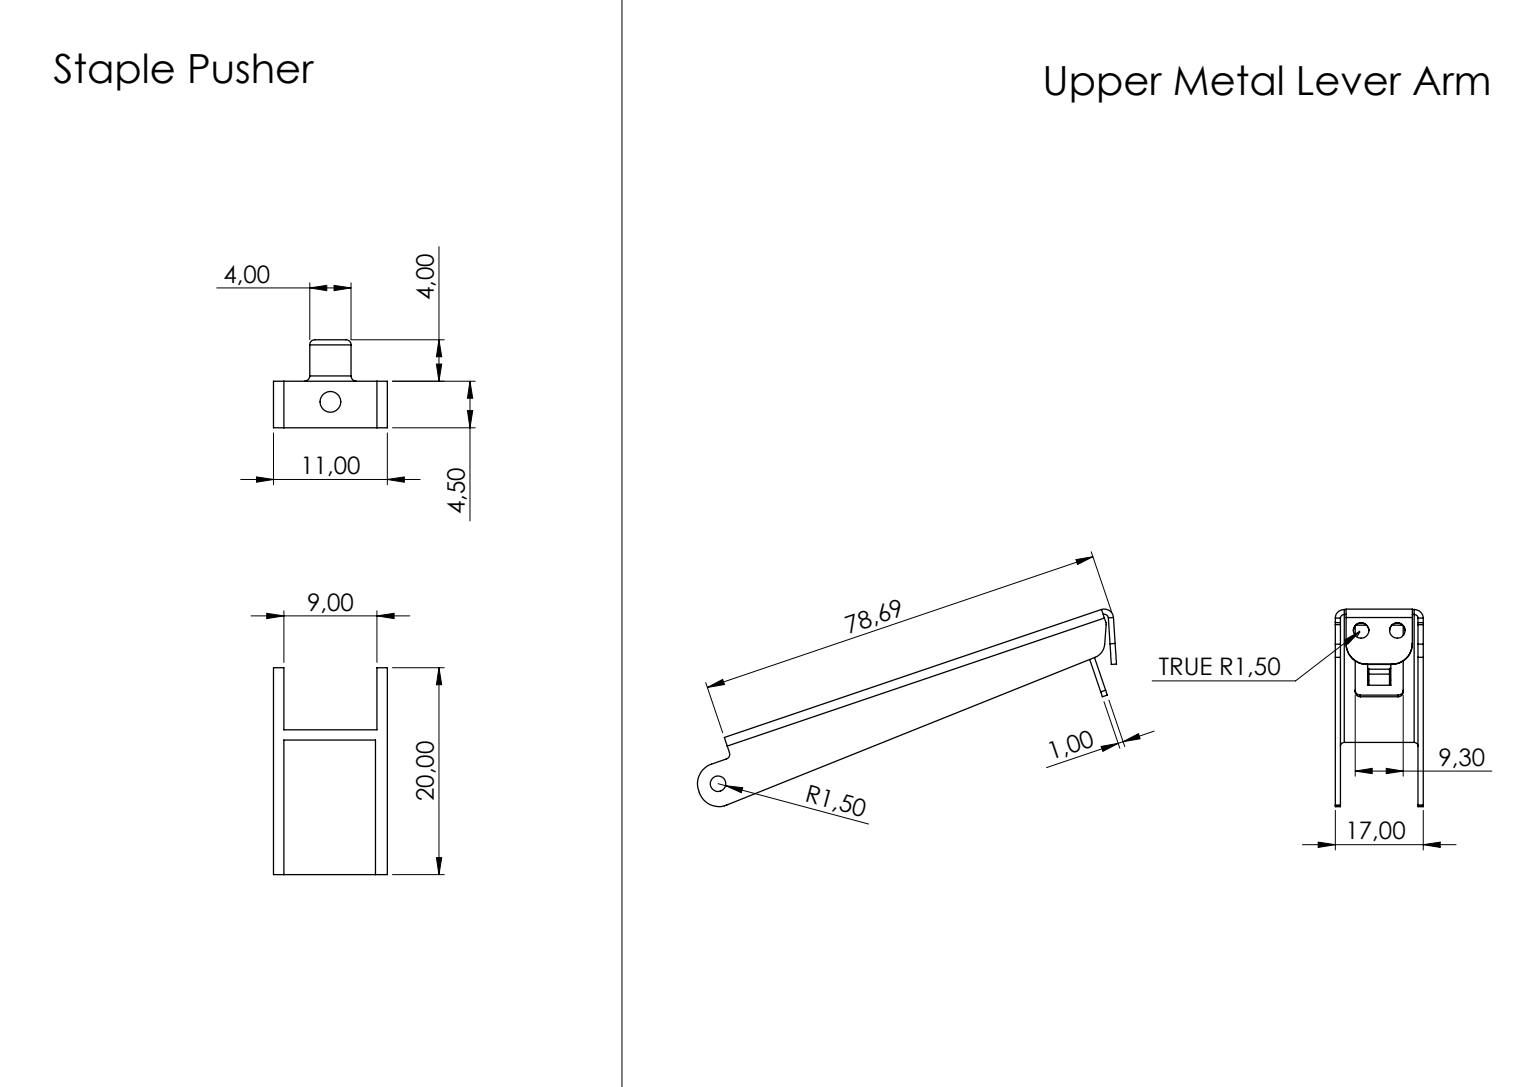
ISO-10303-21;
HEADER;
FILE_DESCRIPTION (('STEP AP214'),
    '1' );
FILE_NAME ('Upper Metal Lever Arm.step',
    '2026-10-06T10:23:46',
    ( '' ),
    ( '' ),
    'SwSTEP 2.0',
    'SolidWorks 2020',
    '' );
FILE_SCHEMA (( 'AUTOMOTIVE_DESIGN' ));
ENDSEC;

DATA;
#3=DIRECTION ( 'NONE',  ( -2.412663730047099099E-15, 0.8967398287344627850, 0.4425581086832399147 ) ) ;
#22=VERTEX_POINT ( 'NONE', #10978 ) ;
#26=DIRECTION ( 'NONE',  ( 1.327674326049719602E-15, -0.4425581086832399147, 0.8967398287344627850 ) ) ;
#34=ORIENTED_EDGE ( 'NONE', *, *, #8349, .T. ) ;
#35=DIRECTION ( 'NONE',  ( -1.000000000000000000, -3.091505625455828697E-15, -4.515976121274772923E-17 ) ) ;
#50=DIRECTION ( 'NONE',  ( 1.000000000000000000, 2.751104698760144965E-15, -1.228345504986737969E-16 ) ) ;
#58=VERTEX_POINT ( 'NONE', #8676 ) ;
#68=EDGE_LOOP ( 'NONE', ( #6538, #19929, #5268, #8723 ) ) ;
#84=CIRCLE ( 'NONE', #17364, 0.7500000000000006661 ) ;
#98=CARTESIAN_POINT ( 'NONE',  ( 29.81606138205697221, -3.227578639999851617, -4.500312080287595329 ) ) ;
#115=ORIENTED_EDGE ( 'NONE', *, *, #16759, .F. ) ;
#117=VECTOR ( 'NONE', #18081, 1000.000000000000000 ) ;
#122=AXIS2_PLACEMENT_3D ( 'NONE', #22603, #19127, #1077 ) ;
#180=VERTEX_POINT ( 'NONE', #7626 ) ;
#184=CARTESIAN_POINT ( 'NONE',  ( 31.91606138205697718, -5.022037326221728826, -5.474317061061731771 ) ) ;
#185=ORIENTED_EDGE ( 'NONE', *, *, #16638, .F. ) ;
#212=VECTOR ( 'NONE', #20996, 1000.000000000000000 ) ;
#213=AXIS2_PLACEMENT_3D ( 'NONE', #12528, #8134, #2696 ) ;
#214=CARTESIAN_POINT ( 'NONE',  ( 33.31606138205700773, -14.32738121993777192, 11.12118157620986558 ) ) ;
#224=ORIENTED_EDGE ( 'NONE', *, *, #10845, .T. ) ;
#227=DIRECTION ( 'NONE',  ( -1.000000000000000000, -2.999999999999999839E-15, 0.000000000000000000 ) ) ;
#238=ORIENTED_EDGE ( 'NONE', *, *, #7921, .F. ) ;
#248=CYLINDRICAL_SURFACE ( 'NONE', #25213, 0.7500000000000006661 ) ;
#274=EDGE_LOOP ( 'NONE', ( #318, #14239, #23744, #24928 ) ) ;
#279=ORIENTED_EDGE ( 'NONE', *, *, #5950, .F. ) ;
#290=ORIENTED_EDGE ( 'NONE', *, *, #14159, .F. ) ;
#298=ORIENTED_EDGE ( 'NONE', *, *, #19568, .F. ) ;
#308=VECTOR ( 'NONE', #6285, 1000.000000000000000 ) ;
#315=ORIENTED_EDGE ( 'NONE', *, *, #21706, .T. ) ;
#318=ORIENTED_EDGE ( 'NONE', *, *, #8973, .F. ) ;
#319=CYLINDRICAL_SURFACE ( 'NONE', #22266, 1.000000000000000888 ) ;
#322=MANIFOLD_SOLID_BREP ( 'NONE', #22112 ) ;
#345=VECTOR ( 'NONE', #23044, 1000.000000000000000 ) ;
#371=LINE ( 'NONE', #16872, #11443 ) ;
#386=CARTESIAN_POINT ( 'NONE',  ( 38.31606138205694378, 4.312150376739274371, 4.986822452676363149 ) ) ;
#387=VECTOR ( 'NONE', #11999, 1000.000000000000000 ) ;
#391=EDGE_CURVE ( 'NONE', #8203, #1835, #13926, .T. ) ;
#405=VECTOR ( 'NONE', #24075, 1000.000000000000000 ) ;
#424=PLANE ( 'NONE',  #3641 ) ;
#427=DIRECTION ( 'NONE',  ( 2.690219486203388234E-15, -0.8967398287344627850, -0.4425581086832399147 ) ) ;
#430=ADVANCED_FACE ( 'NONE', ( #17799 ), #14051, .T. ) ;
#433=CYLINDRICAL_SURFACE ( 'NONE', #4572, 0.7500000000000093259 ) ;
#436=PLANE ( 'NONE',  #12761 ) ;
#445=ORIENTED_EDGE ( 'NONE', *, *, #19266, .F. ) ;
#446=EDGE_CURVE ( 'NONE', #545, #18597, #371, .T. ) ;
#451=CARTESIAN_POINT ( 'NONE',  ( 33.80827534892208064, -18.91453975041207158, 24.37026150481227305 ) ) ;
#452=EDGE_LOOP ( 'NONE', ( #22783, #2146, #1836, #8004 ) ) ;
#459=CARTESIAN_POINT ( 'NONE',  ( 33.66606138205698073, -6.570990706613086374, -2.335727660491067503 ) ) ;
#480=DIRECTION ( 'NONE',  ( 1.327674326049719602E-15, -0.4425581086832399147, 0.8967398287344627850 ) ) ;
#481=AXIS2_PLACEMENT_3D ( 'NONE', #1514, #19059, #7211 ) ;
#483=( NAMED_UNIT ( * ) PLANE_ANGLE_UNIT ( ) SI_UNIT ( $, .RADIAN. ) );
#489=ORIENTED_EDGE ( 'NONE', *, *, #13595, .T. ) ;
#498=VECTOR ( 'NONE', #21104, 1000.000000000000114 ) ;
#502=LINE ( 'NONE', #5275, #212 ) ;
#509=EDGE_CURVE ( 'NONE', #23982, #20593, #22128, .T. ) ;
#523=EDGE_CURVE ( 'NONE', #15010, #2216, #1011, .T. ) ;
#535=ORIENTED_EDGE ( 'NONE', *, *, #15892, .T. ) ;
#545=VERTEX_POINT ( 'NONE', #10703 ) ;
#552=( GEOMETRIC_REPRESENTATION_CONTEXT ( 3 ) GLOBAL_UNCERTAINTY_ASSIGNED_CONTEXT ( ( #3328 ) ) GLOBAL_UNIT_ASSIGNED_CONTEXT ( ( #4972, #12369, #1089 ) ) REPRESENTATION_CONTEXT ( 'NONE', 'WORKASPACE' ) );
#559=VERTEX_POINT ( 'NONE', #14427 ) ;
#561=LINE ( 'NONE', #184, #3329 ) ;
#579=ADVANCED_FACE ( 'NONE', ( #24194 ), #4638, .F. ) ;
#594=EDGE_CURVE ( 'NONE', #6472, #12687, #11972, .T. ) ;
#598=ORIENTED_EDGE ( 'NONE', *, *, #10845, .F. ) ;
#604=ORIENTED_EDGE ( 'NONE', *, *, #15336, .F. ) ;
#611=LINE ( 'NONE', #20075, #6527 ) ;
#612=CARTESIAN_POINT ( 'NONE',  ( 46.81606138205702905, -23.83075694525939170, 32.63712566015296090 ) ) ;
#615=LINE ( 'NONE', #21762, #11077 ) ;
#623=EDGE_CURVE ( 'NONE', #5929, #22719, #8597, .T. ) ;
#628=LINE ( 'NONE', #17704, #1167 ) ;
#645=ORIENTED_EDGE ( 'NONE', *, *, #2860, .F. ) ;
#655=DIRECTION ( 'NONE',  ( -1.000000000000000000, -3.043523379167283935E-15, -1.423844882595663967E-16 ) ) ;
#656=LINE ( 'NONE', #2341, #117 ) ;
#658=EDGE_LOOP ( 'NONE', ( #5985, #10413, #8337, #20417 ) ) ;
#683=LINE ( 'NONE', #22085, #3287 ) ;
#709=CARTESIAN_POINT ( 'NONE',  ( 29.81606138205697221, -3.984974717493133145, -3.847356352999882656 ) ) ;
#710=FACE_OUTER_BOUND ( 'NONE', #21187, .T. ) ;
#714=EDGE_CURVE ( 'NONE', #8686, #3839, #3199, .T. ) ;
#733=DIRECTION ( 'NONE',  ( -1.000000000000000000, -2.999999999999999839E-15, 0.000000000000000000 ) ) ;
#748=ADVANCED_FACE ( 'NONE', ( #710 ), #20321, .F. ) ;
#749=ADVANCED_FACE ( 'NONE', ( #4354 ), #21994, .F. ) ;
#768=DIRECTION ( 'NONE',  ( 0.000000000000000000, -0.4425581086832400257, 0.8967398287344627850 ) ) ;
#776=LINE ( 'NONE', #24468, #17159 ) ;
#780=ORIENTED_EDGE ( 'NONE', *, *, #14281, .T. ) ;
#782=DIRECTION ( 'NONE',  ( -1.000000000000000000, -2.999999999999999839E-15, 0.000000000000000000 ) ) ;
#786=VERTEX_POINT ( 'NONE', #6157 ) ;
#809=CARTESIAN_POINT ( 'NONE',  ( 46.81606138205702194, -20.48383445069734066, 23.59578481461660004 ) ) ;
#834=LINE ( 'NONE', #10778, #14932 ) ;
#863=CARTESIAN_POINT ( 'NONE',  ( 31.91606138205697363, -3.929900956088018038, -7.102449327239662935 ) ) ;
#867=CARTESIAN_POINT ( 'NONE',  ( 42.96606138205694236, 5.208890205473748480, 5.429380561359602453 ) ) ;
#882=FACE_OUTER_BOUND ( 'NONE', #20497, .T. ) ;
#886=ADVANCED_FACE ( 'NONE', ( #3294 ), #4978, .F. ) ;
#896=ORIENTED_EDGE ( 'NONE', *, *, #24579, .T. ) ;
#914=VECTOR ( 'NONE', #23046, 1000.000000000000000 ) ;
#923=DIRECTION ( 'NONE',  ( 2.690219486203388234E-15, -0.8967398287344627850, -0.4425581086832399147 ) ) ;
#925=ORIENTED_EDGE ( 'NONE', *, *, #22452, .T. ) ;
#940=ORIENTED_EDGE ( 'NONE', *, *, #8964, .T. ) ;
#951=FACE_OUTER_BOUND ( 'NONE', #1705, .T. ) ;
#953=DIRECTION ( 'NONE',  ( -1.000000000000000000, -2.999999999999999839E-15, 0.000000000000000000 ) ) ;
#991=DIRECTION ( 'NONE',  ( -4.625929269271484533E-15, 0.8967398287344634511, 0.4425581086832385824 ) ) ;
#992=ORIENTED_EDGE ( 'NONE', *, *, #12189, .F. ) ;
#1011=LINE ( 'NONE', #8894, #24974 ) ;
#1017=EDGE_LOOP ( 'NONE', ( #16280, #22526, #11907, #24276 ) ) ;
#1029=LINE ( 'NONE', #18695, #10688 ) ;
#1034=ADVANCED_FACE ( 'NONE', ( #7294 ), #7553, .T. ) ;
#1043=ADVANCED_FACE ( 'NONE', ( #13603 ), #21202, .T. ) ;
#1047=LINE ( 'NONE', #4925, #6305 ) ;
#1052=DIRECTION ( 'NONE',  ( -2.011972697750612571E-15, 0.6595716529892353686, -0.7516416929448815898 ) ) ;
#1053=ADVANCED_FACE ( 'NONE', ( #5490 ), #11680, .T. ) ;
#1069=FACE_OUTER_BOUND ( 'NONE', #1734, .T. ) ;
#1071=ADVANCED_FACE ( 'NONE', ( #3542 ), #22998, .F. ) ;
#1072=EDGE_CURVE ( 'NONE', #3879, #7931, #5868, .T. ) ;
#1075=VERTEX_POINT ( 'NONE', #13231 ) ;
#1076=CARTESIAN_POINT ( 'NONE',  ( 41.06606138205700063, -13.51824891481308910, 37.72654391001022134 ) ) ;
#1077=DIRECTION ( 'NONE',  ( -4.625929269271484533E-15, 0.8967398287344634511, 0.4425581086832385824 ) ) ;
#1089=( NAMED_UNIT ( * ) SI_UNIT ( $, .STERADIAN. ) SOLID_ANGLE_UNIT ( ) );
#1105=ORIENTED_EDGE ( 'NONE', *, *, #4883, .F. ) ;
#1118=DIRECTION ( 'NONE',  ( 2.011972697750612571E-15, -0.6595716529892353686, 0.7516416929448815898 ) ) ;
#1135=( GEOMETRIC_REPRESENTATION_CONTEXT ( 3 ) GLOBAL_UNCERTAINTY_ASSIGNED_CONTEXT ( ( #17985 ) ) GLOBAL_UNIT_ASSIGNED_CONTEXT ( ( #4006, #12008, #23702 ) ) REPRESENTATION_CONTEXT ( 'NONE', 'WORKASPACE' ) );
#1139=LINE ( 'NONE', #6954, #7217 ) ;
#1156=VERTEX_POINT ( 'NONE', #2386 ) ;
#1157=AXIS2_PLACEMENT_3D ( 'NONE', #10550, #22012, #733 ) ;
#1160=ADVANCED_FACE ( 'NONE', ( #8080 ), #18126, .T. ) ;
#1164=ORIENTED_EDGE ( 'NONE', *, *, #19083, .T. ) ;
#1167=VECTOR ( 'NONE', #35, 1000.000000000000000 ) ;
#1170=DIRECTION ( 'NONE',  ( 1.180247624328911721E-15, -0.3934158747763039088, 0.9193606199277819524 ) ) ;
#1171=CARTESIAN_POINT ( 'NONE',  ( 37.31606138205699352, -10.61256217995208395, 37.48782943861662176 ) ) ;
#1185=LINE ( 'NONE', #1315, #3185 ) ;
#1204=ORIENTED_EDGE ( 'NONE', *, *, #24429, .F. ) ;
#1211=VECTOR ( 'NONE', #15036, 1000.000000000000000 ) ;
#1222=PRESENTATION_STYLE_ASSIGNMENT (( #4371 ) ) ;
#1232=DIRECTION ( 'NONE',  ( 1.000000000000000000, 2.999999999999999839E-15, 0.000000000000000000 ) ) ;
#1238=ORIENTED_EDGE ( 'NONE', *, *, #21451, .T. ) ;
#1254=DIRECTION ( 'NONE',  ( 1.000000000000000000, 3.194449454093636853E-15, 9.596449257708899394E-17 ) ) ;
#1255=EDGE_LOOP ( 'NONE', ( #21618, #11872, #14334, #19616 ) ) ;
#1258=DIRECTION ( 'NONE',  ( 1.327674326049719602E-15, -0.4425581086832399147, 0.8967398287344627850 ) ) ;
#1266=DIRECTION ( 'NONE',  ( -1.327674326049719602E-15, 0.4425581086832399147, -0.8967398287344627850 ) ) ;
#1269=CIRCLE ( 'NONE', #22659, 1.499999999999999778 ) ;
#1274=ADVANCED_FACE ( 'NONE', ( #3147 ), #15131, .T. ) ;
#1278=DIRECTION ( 'NONE',  ( -2.602085213965212219E-15, 0.8967398287344632291, 0.4425581086832389155 ) ) ;
#1285=AXIS2_PLACEMENT_3D ( 'NONE', #5753, #3813, #23012 ) ;
#1287=CYLINDRICAL_SURFACE ( 'NONE', #11276, 3.000000000000000000 ) ;
#1302=EDGE_CURVE ( 'NONE', #5803, #15873, #5351, .T. ) ;
#1315=CARTESIAN_POINT ( 'NONE',  ( 40.31606138205700773, -14.15704008206720843, 14.73030834591676808 ) ) ;
#1320=AXIS2_PLACEMENT_3D ( 'NONE', #1883, #23395, #7445 ) ;
#1344=AXIS2_PLACEMENT_3D ( 'NONE', #22886, #23011, #20710 ) ;
#1355=CARTESIAN_POINT ( 'NONE',  ( 29.81606138205696155, -0.7562224151693598406, -1.633662118351544734 ) ) ;
#1358=LINE ( 'NONE', #13469, #4116 ) ;
#1361=VECTOR ( 'NONE', #5593, 1000.000000000000000 ) ;
#1366=DIRECTION ( 'NONE',  ( 1.225631768639319301E-15, -0.4425581086832399147, 0.8967398287344627850 ) ) ;
#1368=EDGE_CURVE ( 'NONE', #9987, #15268, #10993, .T. ) ;
#1374=LINE ( 'NONE', #5377, #11185 ) ;
#1378=EDGE_CURVE ( 'NONE', #559, #12298, #7156, .T. ) ;
#1384=VECTOR ( 'NONE', #12923, 1000.000000000000000 ) ;
#1396=PLANE ( 'NONE',  #6605 ) ;
#1408=ORIENTED_EDGE ( 'NONE', *, *, #1499, .T. ) ;
#1409=PLANE ( 'NONE',  #22165 ) ;
#1411=DIRECTION ( 'NONE',  ( -1.000000000000000000, -3.091505625455828697E-15, -4.515976121274772923E-17 ) ) ;
#1436=DIRECTION ( 'NONE',  ( 2.792262043613788535E-15, -0.8967398287344627850, -0.4425581086832399147 ) ) ;
#1442=DIRECTION ( 'NONE',  ( -1.327674326049719602E-15, 0.4425581086832399147, -0.8967398287344627850 ) ) ;
#1443=ORIENTED_EDGE ( 'NONE', *, *, #14632, .F. ) ;
#1469=PLANE ( 'NONE',  #4053 ) ;
#1499=EDGE_CURVE ( 'NONE', #17110, #23130, #1965, .T. ) ;
#1514=CARTESIAN_POINT ( 'NONE',  ( 29.81606138205705037, -30.46100403034036219, 72.05704881431053366 ) ) ;
#1522=AXIS2_PLACEMENT_3D ( 'NONE', #25307, #23255, #13610 ) ;
#1527=CARTESIAN_POINT ( 'NONE',  ( 31.91606138205697363, -4.349482454670880571, -5.142398479549302515 ) ) ;
#1532=ORIENTED_EDGE ( 'NONE', *, *, #20926, .F. ) ;
#1535=EDGE_LOOP ( 'NONE', ( #11960, #24521, #19321, #10094 ) ) ;
#1571=EDGE_LOOP ( 'NONE', ( #19061, #21109, #19759, #17406 ) ) ;
#1578=CARTESIAN_POINT ( 'NONE',  ( 36.31606138205702194, -20.02093502212016318, 26.61211107664843212 ) ) ;
#1580=DIRECTION ( 'NONE',  ( -1.000000000000000000, -2.999999999999999839E-15, 0.000000000000000000 ) ) ;
#1594=LINE ( 'NONE', #7420, #2985 ) ;
#1599=CARTESIAN_POINT ( 'NONE',  ( 29.81606138205697221, -3.542416608809870304, -4.744096181734387407 ) ) ;
#1604=CARTESIAN_POINT ( 'NONE',  ( 29.81606138205696155, -0.7562224151693598406, -1.633662118351544734 ) ) ;
#1613=DIRECTION ( 'NONE',  ( 2.690219486203388234E-15, -0.8967398287344627850, -0.4425581086832399147 ) ) ;
#1615=FACE_OUTER_BOUND ( 'NONE', #21424, .T. ) ;
#1619=CIRCLE ( 'NONE', #4529, 0.7500000000000001110 ) ;
#1620=ORIENTED_EDGE ( 'NONE', *, *, #12683, .T. ) ;
#1631=CARTESIAN_POINT ( 'NONE',  ( 29.81606138205697221, -3.542416608809870304, -4.744096181734387407 ) ) ;
#1632=ORIENTED_EDGE ( 'NONE', *, *, #9283, .T. ) ;
#1638=VECTOR ( 'NONE', #3573, 1000.000000000000000 ) ;
#1639=EDGE_LOOP ( 'NONE', ( #23437, #3806, #3552, #24900, #2360, #12605 ) ) ;
#1640=DIRECTION ( 'NONE',  ( -2.312964634635742267E-15, 0.8967398287344634511, 0.4425581086832385824 ) ) ;
#1644=VERTEX_POINT ( 'NONE', #8551 ) ;
#1646=FACE_OUTER_BOUND ( 'NONE', #1724, .T. ) ;
#1647=CARTESIAN_POINT ( 'NONE',  ( 31.91606138205697363, -4.349482454670880571, -5.142398479549302515 ) ) ;
#1651=DIRECTION ( 'NONE',  ( -3.469446951953616555E-15, 0.8967398287344632291, 0.4425581086832389155 ) ) ;
#1659=ORIENTED_EDGE ( 'NONE', *, *, #10742, .T. ) ;
#1667=EDGE_CURVE ( 'NONE', #5253, #2986, #2770, .T. ) ;
#1695=ORIENTED_EDGE ( 'NONE', *, *, #19017, .F. ) ;
#1704=CARTESIAN_POINT ( 'NONE',  ( 45.81606138205697221, -3.984974717493084739, -3.847356352999882656 ) ) ;
#1705=EDGE_LOOP ( 'NONE', ( #1408, #19201, #23703, #1204 ) ) ;
#1706=CYLINDRICAL_SURFACE ( 'NONE', #23794, 1.750000000000001554 ) ;
#1716=CIRCLE ( 'NONE', #3370, 1.499999999999999778 ) ;
#1724=EDGE_LOOP ( 'NONE', ( #1878, #5691, #21493, #16540 ) ) ;
#1728=ADVANCED_FACE ( 'NONE', ( #2604 ), #23989, .F. ) ;
#1729=ORIENTED_EDGE ( 'NONE', *, *, #4047, .T. ) ;
#1734=EDGE_LOOP ( 'NONE', ( #185, #8919, #11633, #24570, #11697, #17570, #604, #9185, #598, #6119, #12537, #16413, #3459 ) ) ;
#1736=DIRECTION ( 'NONE',  ( -1.327674326049719602E-15, 0.4425581086832399147, -0.8967398287344627850 ) ) ;
#1754=DIRECTION ( 'NONE',  ( 3.965082230804126670E-15, -0.8967398287344626739, -0.4425581086832401922 ) ) ;
#1757=DIRECTION ( 'NONE',  ( 1.000000000000000000, 3.091505625455828697E-15, 4.515976121274772923E-17 ) ) ;
#1758=ADVANCED_FACE ( 'NONE', ( #19758 ), #5194, .F. ) ;
#1762=CARTESIAN_POINT ( 'NONE',  ( 34.81606138205697221, -3.103162021984047669, -5.046558096268735305 ) ) ;
#1768=LINE ( 'NONE', #21494, #19414 ) ;
#1778=ORIENTED_EDGE ( 'NONE', *, *, #18713, .F. ) ;
#1785=CIRCLE ( 'NONE', #13752, 3.999999999999997335 ) ;
#1809=DIRECTION ( 'NONE',  ( -1.292451913828718831E-15, 0.4425581086832399147, -0.8967398287344627850 ) ) ;
#1814=CARTESIAN_POINT ( 'NONE',  ( 46.81606138205706458, -34.13844651005145181, 70.48338531520533934 ) ) ;
#1820=EDGE_CURVE ( 'NONE', #24841, #1075, #6741, .T. ) ;
#1824=DIRECTION ( 'NONE',  ( -1.000000000000000000, -2.751104698760144965E-15, 1.228345504986737969E-16 ) ) ;
#1832=CARTESIAN_POINT ( 'NONE',  ( 45.81606138205697221, -3.542416608809821454, -4.744096181734387407 ) ) ;
#1835=VERTEX_POINT ( 'NONE', #11120 ) ;
#1836=ORIENTED_EDGE ( 'NONE', *, *, #15903, .T. ) ;
#1843=LINE ( 'NONE', #23311, #11133 ) ;
#1850=DIRECTION ( 'NONE',  ( 1.133678928659556219E-16, -0.4425581086832399147, 0.8967398287344627850 ) ) ;
#1852=DIRECTION ( 'NONE',  ( -2.690219486203387839E-15, 0.8967398287344625629, 0.4425581086832404143 ) ) ;
#1856=CARTESIAN_POINT ( 'NONE',  ( 40.31606138205699352, -10.61256217995207685, 37.48782943861662886 ) ) ;
#1878=ORIENTED_EDGE ( 'NONE', *, *, #18870, .F. ) ;
#1883=CARTESIAN_POINT ( 'NONE',  ( 41.81606138205696510, -1.316127829577467656, -4.808842309729777220 ) ) ;
#1885=LINE ( 'NONE', #25193, #4850 ) ;
#1888=ORIENTED_EDGE ( 'NONE', *, *, #14158, .T. ) ;
#1897=DIRECTION ( 'NONE',  ( 2.690219486203388234E-15, -0.8967398287344627850, -0.4425581086832399147 ) ) ;
#1904=CARTESIAN_POINT ( 'NONE',  ( 46.81606138205697221, -5.918777154956146980, -5.916875169744970187 ) ) ;
#1918=ORIENTED_EDGE ( 'NONE', *, *, #17611, .F. ) ;
#1923=CIRCLE ( 'NONE', #5236, 1.000000000000000888 ) ;
#1932=FACE_OUTER_BOUND ( 'NONE', #21271, .T. ) ;
#1933=DIRECTION ( 'NONE',  ( -1.327674326049719602E-15, 0.4425581086832399147, -0.8967398287344627850 ) ) ;
#1935=DIRECTION ( 'NONE',  ( -1.000000000000000000, -3.091505625455828697E-15, -4.515976121274772923E-17 ) ) ;
#1939=CARTESIAN_POINT ( 'NONE',  ( 42.96606138205694236, 5.208890205473748480, 5.429380561359602453 ) ) ;
#1959=VERTEX_POINT ( 'NONE', #23203 ) ;
#1965=CIRCLE ( 'NONE', #4849, 1.500000000000000222 ) ;
#1970=ORIENTED_EDGE ( 'NONE', *, *, #10049, .F. ) ;
#1976=DIRECTION ( 'NONE',  ( 1.000000000000000000, 2.751104698760144965E-15, -1.228345504986737969E-16 ) ) ;
#1978=DIRECTION ( 'NONE',  ( 2.341661252633485168E-15, -0.7516416929448815898, -0.6595716529892353686 ) ) ;
#1985=DIRECTION ( 'NONE',  ( -1.000000000000000000, -2.751104698760144965E-15, 1.228345504986737969E-16 ) ) ;
#1994=ORIENTED_EDGE ( 'NONE', *, *, #23549, .T. ) ;
#2000=AXIS2_PLACEMENT_3D ( 'NONE', #9286, #12766, #22537 ) ;
#2002=EDGE_CURVE ( 'NONE', #18170, #19403, #7283, .T. ) ;
#2014=LINE ( 'NONE', #25453, #14717 ) ;
#2022=LINE ( 'NONE', #21993, #11513 ) ;
#2024=CARTESIAN_POINT ( 'NONE',  ( 45.81606138205696510, -3.227578639999803212, -4.500312080287595329 ) ) ;
#2035=CARTESIAN_POINT ( 'NONE',  ( 29.81606138205697221, -3.984974717493133145, -3.847356352999882656 ) ) ;
#2038=EDGE_CURVE ( 'NONE', #7382, #23982, #19598, .T. ) ;
#2051=DIRECTION ( 'NONE',  ( -2.048868001712896742E-15, 0.6595716529892345914, -0.7516416929448823669 ) ) ;
#2062=EDGE_LOOP ( 'NONE', ( #19419, #10057, #1632, #10921 ) ) ;
#2073=DIRECTION ( 'NONE',  ( 1.000000000000000000, 3.091505625455829092E-15, 4.515976121274730398E-17 ) ) ;
#2075=DIRECTION ( 'NONE',  ( -1.000000000000000000, -2.827156040805656045E-15, 8.530177117963464484E-17 ) ) ;
#2077=LINE ( 'NONE', #2210, #20968 ) ;
#2082=CIRCLE ( 'NONE', #6616, 0.7500000000000006661 ) ;
#2086=EDGE_LOOP ( 'NONE', ( #18826, #3522, #1970, #2582 ) ) ;
#2089=AXIS2_PLACEMENT_3D ( 'NONE', #1604, #19524, #1985 ) ;
#2101=VERTEX_POINT ( 'NONE', #25378 ) ;
#2107=EDGE_LOOP ( 'NONE', ( #4877, #14552, #7560, #24954, #3602, #24123 ) ) ;
#2114=EDGE_LOOP ( 'NONE', ( #1105, #6601, #14755, #24647 ) ) ;
#2130=ADVANCED_FACE ( 'NONE', ( #15603 ), #23459, .F. ) ;
#2132=CARTESIAN_POINT ( 'NONE',  ( 33.31606138205700773, -14.32738121993777192, 11.12118157620986558 ) ) ;
#2135=ORIENTED_EDGE ( 'NONE', *, *, #6726, .F. ) ;
#2144=DIRECTION ( 'NONE',  ( -2.312964634635742267E-15, 0.8967398287344634511, 0.4425581086832385824 ) ) ;
#2146=ORIENTED_EDGE ( 'NONE', *, *, #8766, .T. ) ;
#2148=AXIS2_PLACEMENT_3D ( 'NONE', #23261, #1613, #5622 ) ;
#2165=AXIS2_PLACEMENT_3D ( 'NONE', #15015, #24281, #9111 ) ;
#2167=DIRECTION ( 'NONE',  ( 1.000000000000000000, 2.999999999999999839E-15, 0.000000000000000000 ) ) ;
#2172=VECTOR ( 'NONE', #15012, 1000.000000000000000 ) ;
#2179=DIRECTION ( 'NONE',  ( 3.469446951953614189E-15, -0.8967398287344635621, -0.4425581086832386379 ) ) ;
#2210=CARTESIAN_POINT ( 'NONE',  ( 30.81606138205705037, -30.65246816789535345, 72.44500581826353880 ) ) ;
#2216=VERTEX_POINT ( 'NONE', #5988 ) ;
#2220=LINE ( 'NONE', #15877, #21515 ) ;
#2234=CARTESIAN_POINT ( 'NONE',  ( 40.31606138205699352, -9.274586591516573719, 29.12776117315710067 ) ) ;
#2257=DIRECTION ( 'NONE',  ( -1.067465804653198538E-15, 0.4425581086832399147, -0.8967398287344627850 ) ) ;
#2268=FACE_OUTER_BOUND ( 'NONE', #23283, .T. ) ;
#2270=PLANE ( 'NONE',  #24587 ) ;
#2274=VERTEX_POINT ( 'NONE', #23112 ) ;
#2275=EDGE_CURVE ( 'NONE', #18597, #10242, #17586, .T. ) ;
#2285=LINE ( 'NONE', #98, #3817 ) ;
#2287=DIRECTION ( 'NONE',  ( -1.000000000000000000, -2.930207641762116835E-15, -1.414177847953724077E-16 ) ) ;
#2294=LINE ( 'NONE', #14284, #22983 ) ;
#2337=EDGE_LOOP ( 'NONE', ( #22884, #21057, #12205, #7070 ) ) ;
#2341=CARTESIAN_POINT ( 'NONE',  ( 46.81606138205697221, -4.349482454670835274, -5.142398479549302515 ) ) ;
#2344=ADVANCED_FACE ( 'NONE', ( #6238 ), #22329, .F. ) ;
#2360=ORIENTED_EDGE ( 'NONE', *, *, #4498, .F. ) ;
#2370=CARTESIAN_POINT ( 'NONE',  ( 43.31606138205695089, 3.741517323833267294, 2.753690589366190711 ) ) ;
#2379=EDGE_LOOP ( 'NONE', ( #2999, #17890, #19541, #15459 ) ) ;
#2386=CARTESIAN_POINT ( 'NONE',  ( 31.56606138205697576, -5.022037326221730602, -5.474317061061731771 ) ) ;
#2395=AXIS2_PLACEMENT_3D ( 'NONE', #14635, #3156, #12719 ) ;
#2399=DIRECTION ( 'NONE',  ( -4.625929269271484533E-15, 0.8967398287344634511, 0.4425581086832385824 ) ) ;
#2400=CARTESIAN_POINT ( 'NONE',  ( 30.81606138205697931, -5.918777154956195830, -5.916875169744970187 ) ) ;
#2429=ORIENTED_EDGE ( 'NONE', *, *, #14200, .T. ) ;
#2436=VECTOR ( 'NONE', #18030, 1000.000000000000000 ) ;
#2444=FACE_OUTER_BOUND ( 'NONE', #15215, .T. ) ;
#2449=CARTESIAN_POINT ( 'NONE',  ( 40.31606138205697221, -2.780187754385547105, -4.367921789353634843 ) ) ;
#2450=CARTESIAN_POINT ( 'NONE',  ( 40.56606138205696510, -1.522470315718718270, 0.9921758631592225708 ) ) ;
#2453=FACE_OUTER_BOUND ( 'NONE', #3327, .T. ) ;
#2478=ADVANCED_FACE ( 'NONE', ( #2483 ), #10355, .F. ) ;
#2483=FACE_OUTER_BOUND ( 'NONE', #24444, .T. ) ;
#2487=FACE_OUTER_BOUND ( 'NONE', #14398, .T. ) ;
#2512=ORIENTED_EDGE ( 'NONE', *, *, #4337, .T. ) ;
#2514=LINE ( 'NONE', #14380, #3833 ) ;
#2523=CARTESIAN_POINT ( 'NONE',  ( 33.66606138205698073, -6.672912525257930660, -0.4345143786932820218 ) ) ;
#2558=ADVANCED_FACE ( 'NONE', ( #17049 ), #14846, .F. ) ;
#2566=CARTESIAN_POINT ( 'NONE',  ( 45.81606138205707168, -38.42645682328033985, 63.90656833300437256 ) ) ;
#2567=AXIS2_PLACEMENT_3D ( 'NONE', #21845, #11433, #2257 ) ;
#2571=FACE_OUTER_BOUND ( 'NONE', #4228, .T. ) ;
#2582=ORIENTED_EDGE ( 'NONE', *, *, #4044, .F. ) ;
#2586=EDGE_CURVE ( 'NONE', #13895, #14345, #1185, .T. ) ;
#2604=FACE_OUTER_BOUND ( 'NONE', #7979, .T. ) ;
#2623=EDGE_CURVE ( 'NONE', #18307, #12298, #15934, .T. ) ;
#2625=VERTEX_POINT ( 'NONE', #23461 ) ;
#2649=ADVANCED_FACE ( 'NONE', ( #17680 ), #17299, .F. ) ;
#2670=DIRECTION ( 'NONE',  ( 1.000000000000000000, 3.021713267217945694E-15, 1.865775460081201246E-16 ) ) ;
#2696=DIRECTION ( 'NONE',  ( 2.690219486203388234E-15, -0.8967398287344627850, -0.4425581086832399147 ) ) ;
#2698=CARTESIAN_POINT ( 'NONE',  ( 44.71606138205697079, -3.195232061939673240, -6.457771442202879797 ) ) ;
#2704=CARTESIAN_POINT ( 'NONE',  ( 43.31606138205695089, 3.741517323833267294, 2.753690589366190711 ) ) ;
#2709=ORIENTED_EDGE ( 'NONE', *, *, #24840, .F. ) ;
#2722=DIRECTION ( 'NONE',  ( -1.047880217021202589E-15, 0.4425581086832399147, -0.8967398287344627850 ) ) ;
#2738=VERTEX_POINT ( 'NONE', #23593 ) ;
#2746=ORIENTED_EDGE ( 'NONE', *, *, #9299, .F. ) ;
#2748=DIRECTION ( 'NONE',  ( 2.690219486203388234E-15, -0.8967398287344627850, -0.4425581086832399147 ) ) ;
#2753=VECTOR ( 'NONE', #14063, 1000.000000000000000 ) ;
#2758=VERTEX_POINT ( 'NONE', #23205 ) ;
#2762=ADVANCED_FACE ( 'NONE', ( #15740 ), #5572, .T. ) ;
#2767=AXIS2_PLACEMENT_3D ( 'NONE', #14668, #24569, #10568 ) ;
#2770=CIRCLE ( 'NONE', #8983, 1.499999999999994005 ) ;
#2772=DIRECTION ( 'NONE',  ( 1.958867181863079949E-15, -0.6529557272876933549, -0.7573960774932753104 ) ) ;
#2775=CARTESIAN_POINT ( 'NONE',  ( 31.91606138205697363, -3.195232061939711432, -6.457771442202879797 ) ) ;
#2786=EDGE_CURVE ( 'NONE', #786, #13108, #25255, .T. ) ;
#2788=CARTESIAN_POINT ( 'NONE',  ( 31.56606138205697576, -4.349482454670882348, -5.142398479549302515 ) ) ;
#2796=CARTESIAN_POINT ( 'NONE',  ( 46.81606138205705037, -30.65246816789532502, 72.44500581826358143 ) ) ;
#2800=CARTESIAN_POINT ( 'NONE',  ( 44.71606138205697079, -3.854803714928911607, -5.706129749257958572 ) ) ;
#2805=CARTESIAN_POINT ( 'NONE',  ( 36.06606138205696510, -1.522470315718732037, 0.9921758631592225708 ) ) ;
#2823=CIRCLE ( 'NONE', #8627, 3.999999999999997335 ) ;
#2834=DIRECTION ( 'NONE',  ( 0.000000000000000000, -0.7516416929448823669, -0.6595716529892345914 ) ) ;
#2844=DIRECTION ( 'NONE',  ( 2.758081859783345370E-15, -0.9193606199277819524, -0.3934158747763039088 ) ) ;
#2847=VECTOR ( 'NONE', #13700, 1000.000000000000114 ) ;
#2860=EDGE_CURVE ( 'NONE', #16500, #2274, #4004, .T. ) ;
#2862=CARTESIAN_POINT ( 'NONE',  ( 33.31606138205695089, 3.741517323833236208, 2.753690589366190711 ) ) ;
#2868=ORIENTED_EDGE ( 'NONE', *, *, #23949, .T. ) ;
#2878=EDGE_CURVE ( 'NONE', #58, #2101, #22169, .T. ) ;
#2880=VERTEX_POINT ( 'NONE', #16357 ) ;
#2899=CARTESIAN_POINT ( 'NONE',  ( 34.81606138205696510, -1.316127829577488528, -4.808842309729777220 ) ) ;
#2905=CIRCLE ( 'NONE', #4160, 1.750000000000001554 ) ;
#2906=VERTEX_POINT ( 'NONE', #9952 ) ;
#2909=CARTESIAN_POINT ( 'NONE',  ( 46.81606138205697221, -5.022037326221683529, -5.474317061061731771 ) ) ;
#2918=DIRECTION ( 'NONE',  ( 2.690219486203388234E-15, -0.8967398287344627850, -0.4425581086832399147 ) ) ;
#2919=CARTESIAN_POINT ( 'NONE',  ( 29.81606138205706458, -34.13844651005150155, 70.48338531520533934 ) ) ;
#2923=CARTESIAN_POINT ( 'NONE',  ( 34.81606138205696510, -0.8482369431493941292, -3.067843137301039302 ) ) ;
#2932=ORIENTED_EDGE ( 'NONE', *, *, #16638, .T. ) ;
#2933=ORIENTED_EDGE ( 'NONE', *, *, #22167, .F. ) ;
#2959=ORIENTED_EDGE ( 'NONE', *, *, #22645, .T. ) ;
#2974=CIRCLE ( 'NONE', #15738, 0.7499999999999996669 ) ;
#2976=CARTESIAN_POINT ( 'NONE',  ( 43.31606138205700063, -14.32738121993773994, 11.12118157620986558 ) ) ;
#2984=DIRECTION ( 'NONE',  ( 1.327674326049719602E-15, -0.4425581086832399147, 0.8967398287344627850 ) ) ;
#2985=VECTOR ( 'NONE', #17332, 1000.000000000000000 ) ;
#2986=VERTEX_POINT ( 'NONE', #10083 ) ;
#2999=ORIENTED_EDGE ( 'NONE', *, *, #1378, .T. ) ;
#3031=CIRCLE ( 'NONE', #18669, 3.999999999999997335 ) ;
#3039=DIRECTION ( 'NONE',  ( -1.327674326049719602E-15, 0.4425581086832399147, -0.8967398287344627850 ) ) ;
#3041=( GEOMETRIC_REPRESENTATION_CONTEXT ( 3 ) GLOBAL_UNCERTAINTY_ASSIGNED_CONTEXT ( ( #24699 ) ) GLOBAL_UNIT_ASSIGNED_CONTEXT ( ( #5109, #483, #22135 ) ) REPRESENTATION_CONTEXT ( 'NONE', 'WORKASPACE' ) );
#3045=FACE_OUTER_BOUND ( 'NONE', #25037, .T. ) ;
#3063=ORIENTED_EDGE ( 'NONE', *, *, #3083, .T. ) ;
#3068=ORIENTED_EDGE ( 'NONE', *, *, #18672, .T. ) ;
#3072=LINE ( 'NONE', #5016, #12394 ) ;
#3074=DIRECTION ( 'NONE',  ( 1.000000000000000000, 2.602085213965208275E-15, 0.000000000000000000 ) ) ;
#3083=EDGE_CURVE ( 'NONE', #4595, #4703, #12650, .T. ) ;
#3089=EDGE_CURVE ( 'NONE', #2986, #5253, #14766, .T. ) ;
#3106=EDGE_CURVE ( 'NONE', #15655, #12192, #22421, .T. ) ;
#3107=ORIENTED_EDGE ( 'NONE', *, *, #18870, .T. ) ;
#3120=ORIENTED_EDGE ( 'NONE', *, *, #12244, .F. ) ;
#3122=CARTESIAN_POINT ( 'NONE',  ( 35.91606138205695942, 0.5799492015812600654, -3.145019409304214530 ) ) ;
#3134=ORIENTED_EDGE ( 'NONE', *, *, #5824, .F. ) ;
#3139=ORIENTED_EDGE ( 'NONE', *, *, #5484, .T. ) ;
#3141=CARTESIAN_POINT ( 'NONE',  ( 46.81606138205696510, -2.286980848581572356, -4.124514829577853980 ) ) ;
#3142=DIRECTION ( 'NONE',  ( 1.000000000000000000, 2.999999999999999839E-15, 0.000000000000000000 ) ) ;
#3144=CARTESIAN_POINT ( 'NONE',  ( 45.81606138205705037, -30.65246816789533213, 72.44500581826358143 ) ) ;
#3147=FACE_OUTER_BOUND ( 'NONE', #2379, .T. ) ;
#3148=ORIENTED_EDGE ( 'NONE', *, *, #12027, .F. ) ;
#3156=DIRECTION ( 'NONE',  ( -2.048868001712898319E-15, 0.6595716529892350355, -0.7516416929448821449 ) ) ;
#3166=ORIENTED_EDGE ( 'NONE', *, *, #10381, .T. ) ;
#3181=ORIENTED_EDGE ( 'NONE', *, *, #23246, .F. ) ;
#3185=VECTOR ( 'NONE', #8688, 1000.000000000000000 ) ;
#3190=EDGE_CURVE ( 'NONE', #22354, #4595, #18463, .T. ) ;
#3193=LINE ( 'NONE', #24443, #13204 ) ;
#3199=CIRCLE ( 'NONE', #12271, 1.500000000000000222 ) ;
#3202=EDGE_LOOP ( 'NONE', ( #12001, #23376, #21364, #9011 ) ) ;
#3204=DIRECTION ( 'NONE',  ( 1.000000000000000000, 2.611101091812726599E-15, -1.919289851541777660E-16 ) ) ;
#3217=VECTOR ( 'NONE', #23669, 1000.000000000000000 ) ;
#3223=CARTESIAN_POINT ( 'NONE',  ( 46.81606138205696510, -3.028410647649130816, 0.3252050635115383281 ) ) ;
#3250=EDGE_CURVE ( 'NONE', #8203, #1959, #4071, .T. ) ;
#3259=VECTOR ( 'NONE', #4287, 1000.000000000000000 ) ;
#3268=VERTEX_POINT ( 'NONE', #13655 ) ;
#3274=DIRECTION ( 'NONE',  ( -2.690219486203388234E-15, 0.8967398287344627850, 0.4425581086832399147 ) ) ;
#3287=VECTOR ( 'NONE', #16155, 1000.000000000000000 ) ;
#3294=FACE_OUTER_BOUND ( 'NONE', #4552, .T. ) ;
#3302=DIRECTION ( 'NONE',  ( 0.000000000000000000, -0.4425581086832348077, 0.8967398287344653385 ) ) ;
#3305=ORIENTED_EDGE ( 'NONE', *, *, #5617, .T. ) ;
#3313=VECTOR ( 'NONE', #7589, 1000.000000000000000 ) ;
#3319=CARTESIAN_POINT ( 'NONE',  ( 35.91606138205694521, 3.586515973360777654, -0.5067327973472466329 ) ) ;
#3325=DIRECTION ( 'NONE',  ( -1.000000000000000000, -2.999999999999999839E-15, 0.000000000000000000 ) ) ;
#3327=EDGE_LOOP ( 'NONE', ( #12452, #6895, #16216, #13853 ) ) ;
#3328=UNCERTAINTY_MEASURE_WITH_UNIT (LENGTH_MEASURE( 1.000000000000000082E-05 ), #4972, 'distance_accuracy_value', 'NONE');
#3329=VECTOR ( 'NONE', #7940, 1000.000000000000000 ) ;
#3355=ORIENTED_EDGE ( 'NONE', *, *, #9648, .T. ) ;
#3358=CARTESIAN_POINT ( 'NONE',  ( 33.31606138205697931, -6.570990706613088150, -2.335727660491067503 ) ) ;
#3367=EDGE_LOOP ( 'NONE', ( #25040, #9996, #22376, #20015 ) ) ;
#3369=LINE ( 'NONE', #1171, #6711 ) ;
#3370=AXIS2_PLACEMENT_3D ( 'NONE', #9033, #24457, #6829 ) ;
#3380=CIRCLE ( 'NONE', #10783, 1.750000000000001554 ) ;
#3386=ADVANCED_FACE ( 'NONE', ( #23808 ), #9923, .T. ) ;
#3407=EDGE_CURVE ( 'NONE', #2216, #7931, #18892, .T. ) ;
#3424=LINE ( 'NONE', #17090, #22197 ) ;
#3428=VECTOR ( 'NONE', #14336, 1000.000000000000000 ) ;
#3429=LINE ( 'NONE', #25165, #3725 ) ;
#3431=VERTEX_POINT ( 'NONE', #17780 ) ;
#3433=CARTESIAN_POINT ( 'NONE',  ( 40.31606138205697931, -5.528433326023618477, -4.448224773462933435 ) ) ;
#3442=EDGE_CURVE ( 'NONE', #58, #1644, #2294, .T. ) ;
#3444=AXIS2_PLACEMENT_3D ( 'NONE', #19832, #8112, #10052 ) ;
#3452=LINE ( 'NONE', #13629, #9000 ) ;
#3459=ORIENTED_EDGE ( 'NONE', *, *, #7029, .F. ) ;
#3463=LINE ( 'NONE', #6724, #9559 ) ;
#3486=EDGE_CURVE ( 'NONE', #21683, #5803, #615, .T. ) ;
#3491=DIRECTION ( 'NONE',  ( -2.011972697750612571E-15, 0.6595716529892353686, -0.7516416929448815898 ) ) ;
#3493=SURFACE_STYLE_FILL_AREA ( #19094 ) ;
#3495=FACE_OUTER_BOUND ( 'NONE', #2062, .T. ) ;
#3505=CARTESIAN_POINT ( 'NONE',  ( 44.71606138205695657, 0.5799492015812843793, -3.145019409304214530 ) ) ;
#3522=ORIENTED_EDGE ( 'NONE', *, *, #2038, .F. ) ;
#3526=CARTESIAN_POINT ( 'NONE',  ( 30.81606138205694378, 5.290470704224592424, -0.3848988112044732235 ) ) ;
#3538=CARTESIAN_POINT ( 'NONE',  ( 45.81606138205707168, -36.80651332587431313, 65.82119181171029254 ) ) ;
#3542=FACE_OUTER_BOUND ( 'NONE', #19197, .T. ) ;
#3552=ORIENTED_EDGE ( 'NONE', *, *, #1378, .F. ) ;
#3555=FACE_OUTER_BOUND ( 'NONE', #11528, .T. ) ;
#3561=CARTESIAN_POINT ( 'NONE',  ( 30.81606138205707168, -37.26069504592557990, 64.48189387429259511 ) ) ;
#3562=DIRECTION ( 'NONE',  ( -1.000000000000000000, -2.999999999999999839E-15, 0.000000000000000000 ) ) ;
#3565=AXIS2_PLACEMENT_3D ( 'NONE', #1856, #23499, #13357 ) ;
#3571=EDGE_CURVE ( 'NONE', #11586, #20804, #22520, .T. ) ;
#3573=DIRECTION ( 'NONE',  ( 1.000000000000000000, 2.751104698760144965E-15, -1.228345504986737969E-16 ) ) ;
#3589=CARTESIAN_POINT ( 'NONE',  ( 35.56606138205702194, -20.30191568716149675, 23.22716926412510219 ) ) ;
#3593=CARTESIAN_POINT ( 'NONE',  ( 45.81606138205707879, -39.99575152356564445, 63.13209164280871022 ) ) ;
#3602=ORIENTED_EDGE ( 'NONE', *, *, #20581, .F. ) ;
#3603=VECTOR ( 'NONE', #20223, 1000.000000000000000 ) ;
#3609=ORIENTED_EDGE ( 'NONE', *, *, #8349, .F. ) ;
#3612=SURFACE_STYLE_USAGE ( .BOTH. , #25107 ) ;
#3630=CARTESIAN_POINT ( 'NONE',  ( 46.81606138205707168, -38.13418765192403015, 68.51141129791366780 ) ) ;
#3639=AXIS2_PLACEMENT_3D ( 'NONE', #5279, #9032, #24576 ) ;
#3641=AXIS2_PLACEMENT_3D ( 'NONE', #13847, #4440, #7932 ) ;
#3662=VECTOR ( 'NONE', #11484, 1000.000000000000000 ) ;
#3664=FACE_OUTER_BOUND ( 'NONE', #19556, .T. ) ;
#3665=DIRECTION ( 'NONE',  ( -2.574571254471601357E-15, 0.8967398287344627850, 0.4425581086832399147 ) ) ;
#3666=DIRECTION ( 'NONE',  ( -1.000000000000000000, -2.999999999999999839E-15, 0.000000000000000000 ) ) ;
#3687=DIRECTION ( 'NONE',  ( 1.000000000000000000, 3.965082230804126670E-15, 0.000000000000000000 ) ) ;
#3695=AXIS2_PLACEMENT_3D ( 'NONE', #8825, #18351, #4943 ) ;
#3701=CARTESIAN_POINT ( 'NONE',  ( 30.81606138205706458, -34.54722833698622964, 70.28164373264664277 ) ) ;
#3705=CARTESIAN_POINT ( 'NONE',  ( 45.81606138205695800, -0.2703287878657676391, 1.505452687840413972 ) ) ;
#3709=CARTESIAN_POINT ( 'NONE',  ( 29.81606138205706458, -34.55876147768187678, 70.30501292735635843 ) ) ;
#3725=VECTOR ( 'NONE', #17094, 1000.000000000000000 ) ;
#3731=CARTESIAN_POINT ( 'NONE',  ( 41.81606138205696510, -1.975699482566714904, -4.057200616784870206 ) ) ;
#3743=CYLINDRICAL_SURFACE ( 'NONE', #22838, 1.000000000000000000 ) ;
#3747=PLANE ( 'NONE',  #8647 ) ;
#3753=ORIENTED_EDGE ( 'NONE', *, *, #23120, .F. ) ;
#3754=ADVANCED_FACE ( 'NONE', ( #25456, #7834, #17885 ), #5898, .T. ) ;
#3757=PRODUCT_CONTEXT ( 'NONE', #22302, 'mechanical' ) ;
#3772=ORIENTED_EDGE ( 'NONE', *, *, #6897, .T. ) ;
#3806=ORIENTED_EDGE ( 'NONE', *, *, #2623, .T. ) ;
#3813=DIRECTION ( 'NONE',  ( -1.000000000000000000, -2.999999999999999839E-15, 0.000000000000000000 ) ) ;
#3817=VECTOR ( 'NONE', #19823, 1000.000000000000000 ) ;
#3819=ORIENTED_EDGE ( 'NONE', *, *, #16170, .T. ) ;
#3824=ADVANCED_FACE ( 'NONE', ( #11597 ), #15319, .T. ) ;
#3833=VECTOR ( 'NONE', #19930, 1000.000000000000000 ) ;
#3839=VERTEX_POINT ( 'NONE', #13401 ) ;
#3851=CARTESIAN_POINT ( 'NONE',  ( 46.81606138205697221, -3.984974717493081187, -3.847356352999882656 ) ) ;
#3865=CIRCLE ( 'NONE', #7581, 1.000000000000011990 ) ;
#3875=EDGE_CURVE ( 'NONE', #21859, #2986, #23169, .T. ) ;
#3879=VERTEX_POINT ( 'NONE', #21248 ) ;
#3901=ADVANCED_FACE ( 'NONE', ( #1646 ), #9539, .T. ) ;
#3932=EDGE_CURVE ( 'NONE', #7931, #1075, #25345, .T. ) ;
#3934=CARTESIAN_POINT ( 'NONE',  ( 45.06606138205697221, -5.022037326221688858, -5.474317061061731771 ) ) ;
#3940=DIRECTION ( 'NONE',  ( -1.327674326049719602E-15, 0.4425581086832399147, -0.8967398287344627850 ) ) ;
#3978=ORIENTED_EDGE ( 'NONE', *, *, #13595, .F. ) ;
#3980=CARTESIAN_POINT ( 'NONE',  ( 31.56606138205707879, -39.09901169483120498, 63.57464975149190423 ) ) ;
#3987=CARTESIAN_POINT ( 'NONE',  ( 45.06606138205707879, -38.42645682328033985, 63.90656833300437256 ) ) ;
#3991=CARTESIAN_POINT ( 'NONE',  ( 29.81606138205709300, -43.53621639303161572, 70.30601027268440362 ) ) ;
#3996=EDGE_CURVE ( 'NONE', #7231, #14345, #8614, .T. ) ;
#4004=CIRCLE ( 'NONE', #18821, 0.7499999999999985567 ) ;
#4006=( LENGTH_UNIT ( ) NAMED_UNIT ( * ) SI_UNIT ( .MILLI., .METRE. ) );
#4007=ORIENTED_EDGE ( 'NONE', *, *, #14159, .T. ) ;
#4022=DIRECTION ( 'NONE',  ( -2.574571254471601357E-15, 0.8967398287344627850, 0.4425581086832399147 ) ) ;
#4024=DIRECTION ( 'NONE',  ( 0.000000000000000000, 0.6595716529892349245, -0.7516416929448820339 ) ) ;
#4033=ORIENTED_EDGE ( 'NONE', *, *, #3407, .T. ) ;
#4044=EDGE_CURVE ( 'NONE', #20593, #18694, #9123, .T. ) ;
#4047=EDGE_CURVE ( 'NONE', #13742, #19743, #12850, .T. ) ;
#4053=AXIS2_PLACEMENT_3D ( 'NONE', #3526, #3274, #1580 ) ;
#4071=CIRCLE ( 'NONE', #23396, 1.000000000000000000 ) ;
#4080=AXIS2_PLACEMENT_3D ( 'NONE', #20303, #18610, #953 ) ;
#4088=VECTOR ( 'NONE', #14601, 1000.000000000000000 ) ;
#4098=CARTESIAN_POINT ( 'NONE',  ( 41.06606138205700063, -13.51824891481308910, 37.72654391001022134 ) ) ;
#4103=ORIENTED_EDGE ( 'NONE', *, *, #5014, .F. ) ;
#4107=ORIENTED_EDGE ( 'NONE', *, *, #1499, .F. ) ;
#4113=CARTESIAN_POINT ( 'NONE',  ( 36.31606138205696510, -2.780187754385557319, -4.367921789353634843 ) ) ;
#4116=VECTOR ( 'NONE', #3665, 1000.000000000000000 ) ;
#4118=DIRECTION ( 'NONE',  ( 0.000000000000000000, -0.4425581086832385824, 0.8967398287344634511 ) ) ;
#4122=DIRECTION ( 'NONE',  ( 2.792262043613788535E-15, -0.8967398287344627850, -0.4425581086832399147 ) ) ;
#4129=CARTESIAN_POINT ( 'NONE',  ( 34.81606138205695800, -0.1886652901601799104, -3.819484830245897911 ) ) ;
#4136=CARTESIAN_POINT ( 'NONE',  ( 46.81606138205697221, -3.542416608809818346, -4.744096181734387407 ) ) ;
#4157=LINE ( 'NONE', #8275, #20131 ) ;
#4160=AXIS2_PLACEMENT_3D ( 'NONE', #24016, #12704, #6391 ) ;
#4167=AXIS2_PLACEMENT_3D ( 'NONE', #19645, #15654, #9368 ) ;
#4172=CYLINDRICAL_SURFACE ( 'NONE', #10075, 1.000000000000000888 ) ;
#4191=VERTEX_POINT ( 'NONE', #12193 ) ;
#4193=ORIENTED_EDGE ( 'NONE', *, *, #8608, .T. ) ;
#4207=EDGE_CURVE ( 'NONE', #15653, #24211, #683, .T. ) ;
#4215=EDGE_CURVE ( 'NONE', #22990, #1075, #18114, .T. ) ;
#4218=ORIENTED_EDGE ( 'NONE', *, *, #23120, .T. ) ;
#4220=DIRECTION ( 'NONE',  ( -2.792262043613788535E-15, 0.8967398287344627850, 0.4425581086832399147 ) ) ;
#4221=AXIS2_PLACEMENT_3D ( 'NONE', #18915, #4872, #1258 ) ;
#4228=EDGE_LOOP ( 'NONE', ( #18609, #19894, #8711, #23244 ) ) ;
#4229=CARTESIAN_POINT ( 'NONE',  ( 40.56606138205696510, -1.965028424401960461, 1.888915691893686244 ) ) ;
#4231=ADVANCED_FACE ( 'NONE', ( #4449 ), #436, .T. ) ;
#4238=EDGE_CURVE ( 'NONE', #12829, #6472, #1619, .T. ) ;
#4242=CIRCLE ( 'NONE', #21156, 1.500000000000000222 ) ;
#4248=ADVANCED_FACE ( 'NONE', ( #12578 ), #10372, .F. ) ;
#4253=DIRECTION ( 'NONE',  ( -2.792262043613788535E-15, 0.8967398287344627850, 0.4425581086832398592 ) ) ;
#4255=ORIENTED_EDGE ( 'NONE', *, *, #24177, .T. ) ;
#4261=ORIENTED_EDGE ( 'NONE', *, *, #5484, .F. ) ;
#4262=AXIS2_PLACEMENT_3D ( 'NONE', #18101, #10114, #12305 ) ;
#4273=CARTESIAN_POINT ( 'NONE',  ( 29.81606138205707168, -36.80651332587436286, 65.82119181171029254 ) ) ;
#4287=DIRECTION ( 'NONE',  ( -2.792262043613788535E-15, 0.8967398287344627850, 0.4425581086832399147 ) ) ;
#4295=ORIENTED_EDGE ( 'NONE', *, *, #23106, .T. ) ;
#4296=CARTESIAN_POINT ( 'NONE',  ( 30.81606138205707524, -38.42645682328038248, 63.90656833300437256 ) ) ;
#4297=AXIS2_PLACEMENT_3D ( 'NONE', #15497, #7785, #7912 ) ;
#4310=DIRECTION ( 'NONE',  ( -1.000000000000000000, -2.999999999999999839E-15, 0.000000000000000000 ) ) ;
#4312=DIRECTION ( 'NONE',  ( 1.327674326049719602E-15, -0.4425581086832399147, 0.8967398287344627850 ) ) ;
#4325=ORIENTED_EDGE ( 'NONE', *, *, #4714, .T. ) ;
#4326=DIRECTION ( 'NONE',  ( -1.000000000000000000, -2.999999999999999839E-15, 0.000000000000000000 ) ) ;
#4329=DIRECTION ( 'NONE',  ( -1.327674326049719602E-15, 0.4425581086832399147, -0.8967398287344627850 ) ) ;
#4337=EDGE_CURVE ( 'NONE', #23131, #16929, #20031, .T. ) ;
#4346=DIRECTION ( 'NONE',  ( 1.000000000000000000, 2.999999999999999839E-15, 0.000000000000000000 ) ) ;
#4349=DIRECTION ( 'NONE',  ( -1.000000000000000000, -2.999999999999999839E-15, 0.000000000000000000 ) ) ;
#4354=FACE_OUTER_BOUND ( 'NONE', #14705, .T. ) ;
#4362=CARTESIAN_POINT ( 'NONE',  ( 45.81606138205696510, -3.028410647649132592, 0.3252050635115383281 ) ) ;
#4364=CARTESIAN_POINT ( 'NONE',  ( 46.81606138205701484, -19.34838015056928029, 26.94402965816085072 ) ) ;
#4367=CARTESIAN_POINT ( 'NONE',  ( 40.31606138205701484, -18.91453975041205382, 24.37026150481227305 ) ) ;
#4371=SURFACE_STYLE_USAGE ( .BOTH. , #16693 ) ;
#4390=CARTESIAN_POINT ( 'NONE',  ( 46.81606138205695800, -0.7562224151693112129, -1.633662118351544734 ) ) ;
#4404=LINE ( 'NONE', #20115, #5273 ) ;
#4417=ORIENTED_EDGE ( 'NONE', *, *, #8727, .T. ) ;
#4419=CYLINDRICAL_SURFACE ( 'NONE', #7963, 1.750000000000001998 ) ;
#4424=CARTESIAN_POINT ( 'NONE',  ( 44.71606138205697079, -3.854803714928911607, -5.706129749257958572 ) ) ;
#4430=EDGE_CURVE ( 'NONE', #4703, #9931, #13981, .T. ) ;
#4434=AXIS2_PLACEMENT_3D ( 'NONE', #21593, #3940, #21713 ) ;
#4440=DIRECTION ( 'NONE',  ( -2.792262043613788535E-15, 0.8967398287344627850, 0.4425581086832399147 ) ) ;
#4449=FACE_OUTER_BOUND ( 'NONE', #15155, .T. ) ;
#4456=EDGE_LOOP ( 'NONE', ( #21260, #25077, #17488, #8737 ) ) ;
#4474=DIRECTION ( 'NONE',  ( -1.271715504244016160E-15, 0.4425581086832399147, -0.8967398287344627850 ) ) ;
#4475=VECTOR ( 'NONE', #14510, 1000.000000000000000 ) ;
#4485=CARTESIAN_POINT ( 'NONE',  ( 40.71606138205695657, 2.926944320371565045, 0.2449088955976189141 ) ) ;
#4492=DIRECTION ( 'NONE',  ( -1.000000000000000000, -3.091505625455828697E-15, -4.515976121274771690E-17 ) ) ;
#4498=EDGE_CURVE ( 'NONE', #12192, #786, #15492, .T. ) ;
#4502=VECTOR ( 'NONE', #4022, 1000.000000000000000 ) ;
#4505=DIRECTION ( 'NONE',  ( 0.000000000000000000, 0.8967398287344635621, 0.4425581086832386379 ) ) ;
#4513=VECTOR ( 'NONE', #16714, 1000.000000000000000 ) ;
#4517=ORIENTED_EDGE ( 'NONE', *, *, #24579, .F. ) ;
#4529=AXIS2_PLACEMENT_3D ( 'NONE', #12316, #6626, #20162 ) ;
#4532=EDGE_CURVE ( 'NONE', #3879, #19656, #9968, .T. ) ;
#4534=AXIS2_PLACEMENT_3D ( 'NONE', #10560, #14543, #2179 ) ;
#4552=EDGE_LOOP ( 'NONE', ( #22053, #24111, #23848, #23752 ) ) ;
#4572=AXIS2_PLACEMENT_3D ( 'NONE', #23641, #4326, #8185 ) ;
#4588=LINE ( 'NONE', #12455, #19435 ) ;
#4592=ORIENTED_EDGE ( 'NONE', *, *, #2878, .T. ) ;
#4595=VERTEX_POINT ( 'NONE', #23609 ) ;
#4596=DIRECTION ( 'NONE',  ( 3.965082230804126670E-15, -0.8967398287344626739, -0.4425581086832401922 ) ) ;
#4605=LINE ( 'NONE', #2400, #16058 ) ;
#4617=PLANE ( 'NONE',  #13281 ) ;
#4621=LINE ( 'NONE', #612, #14507 ) ;
#4622=CARTESIAN_POINT ( 'NONE',  ( 31.91606138205695942, 0.5799492015812461876, -3.145019409304214530 ) ) ;
#4627=ORIENTED_EDGE ( 'NONE', *, *, #8386, .T. ) ;
#4630=DIRECTION ( 'NONE',  ( -1.000000000000000000, -2.999999999999999839E-15, 0.000000000000000000 ) ) ;
#4631=VERTEX_POINT ( 'NONE', #1832 ) ;
#4638=CYLINDRICAL_SURFACE ( 'NONE', #2767, 1.499999999999999778 ) ;
#4649=CARTESIAN_POINT ( 'NONE',  ( 46.81606138205705037, -30.46100403034029114, 72.05704881431049103 ) ) ;
#4675=CARTESIAN_POINT ( 'NONE',  ( 29.81606138205706813, -35.90867894478446232, 74.07034463014319670 ) ) ;
#4676=ADVANCED_FACE ( 'NONE', ( #9465 ), #25394, .T. ) ;
#4694=FACE_BOUND ( 'NONE', #6589, .T. ) ;
#4703=VERTEX_POINT ( 'NONE', #20000 ) ;
#4709=ORIENTED_EDGE ( 'NONE', *, *, #11772, .F. ) ;
#4714=EDGE_CURVE ( 'NONE', #8502, #2738, #24100, .T. ) ;
#4716=DIRECTION ( 'NONE',  ( 1.000000000000000000, 2.999999999999999839E-15, 0.000000000000000000 ) ) ;
#4742=CARTESIAN_POINT ( 'NONE',  ( 42.96606138205694236, 5.651448314156994002, 4.532640732625139002 ) ) ;
#4744=LINE ( 'NONE', #12618, #19308 ) ;
#4778=ADVANCED_FACE ( 'NONE', ( #18331 ), #6355, .T. ) ;
#4779=VERTEX_POINT ( 'NONE', #4296 ) ;
#4785=ORIENTED_EDGE ( 'NONE', *, *, #9687, .F. ) ;
#4786=DIRECTION ( 'NONE',  ( -1.000000000000000000, -2.999999999999999839E-15, 0.000000000000000000 ) ) ;
#4797=DIRECTION ( 'NONE',  ( 0.000000000000000000, -0.4425581086832397482, 0.8967398287344628960 ) ) ;
#4817=DIRECTION ( 'NONE',  ( -1.133678928659556219E-16, 0.4425581086832399147, -0.8967398287344627850 ) ) ;
#4823=CARTESIAN_POINT ( 'NONE',  ( 43.31606138205698642, -7.467730535347520515, -2.778285769174305919 ) ) ;
#4828=AXIS2_PLACEMENT_3D ( 'NONE', #9703, #25379, #25121 ) ;
#4838=ORIENTED_EDGE ( 'NONE', *, *, #23556, .F. ) ;
#4839=DIRECTION ( 'NONE',  ( -1.000000000000000000, -3.469446951953611033E-15, 0.000000000000000000 ) ) ;
#4847=DIRECTION ( 'NONE',  ( -1.000000000000000000, -2.999999999999999839E-15, 0.000000000000000000 ) ) ;
#4849=AXIS2_PLACEMENT_3D ( 'NONE', #23107, #19507, #17201 ) ;
#4850=VECTOR ( 'NONE', #15550, 1000.000000000000000 ) ;
#4863=FACE_BOUND ( 'NONE', #13578, .T. ) ;
#4866=EDGE_CURVE ( 'NONE', #2216, #2880, #7239, .T. ) ;
#4871=FACE_BOUND ( 'NONE', #2107, .T. ) ;
#4872=DIRECTION ( 'NONE',  ( 2.497472433317076378E-15, -0.8967398287344627850, -0.4425581086832399147 ) ) ;
#4877=ORIENTED_EDGE ( 'NONE', *, *, #22949, .F. ) ;
#4883=EDGE_CURVE ( 'NONE', #2906, #22, #18827, .T. ) ;
#4888=ORIENTED_EDGE ( 'NONE', *, *, #7043, .F. ) ;
#4897=LINE ( 'NONE', #7087, #7167 ) ;
#4901=CARTESIAN_POINT ( 'NONE',  ( 45.81606138205706458, -34.55876147768182705, 70.30501292735635843 ) ) ;
#4903=AXIS2_PLACEMENT_3D ( 'NONE', #15152, #16704, #3302 ) ;
#4925=CARTESIAN_POINT ( 'NONE',  ( 33.31606138205697221, -3.118133360756983663, 16.65315793475036443 ) ) ;
#4943=DIRECTION ( 'NONE',  ( -2.690219486203388234E-15, 0.8967398287344627850, 0.4425581086832399147 ) ) ;
#4958=CYLINDRICAL_SURFACE ( 'NONE', #21578, 1.499999999999999778 ) ;
#4959=FACE_OUTER_BOUND ( 'NONE', #22359, .T. ) ;
#4972=( LENGTH_UNIT ( ) NAMED_UNIT ( * ) SI_UNIT ( .MILLI., .METRE. ) );
#4978=PLANE ( 'NONE',  #23783 ) ;
#4981=DIRECTION ( 'NONE',  ( -1.000000000000000000, -2.751104698760144965E-15, 1.228345504986737969E-16 ) ) ;
#5003=ADVANCED_FACE ( 'NONE', ( #8799 ), #5046, .T. ) ;
#5007=VECTOR ( 'NONE', #13679, 1000.000000000000000 ) ;
#5014=EDGE_CURVE ( 'NONE', #8846, #17722, #19587, .T. ) ;
#5016=CARTESIAN_POINT ( 'NONE',  ( 46.81606138205707168, -35.90387122078352178, 69.64117576433150703 ) ) ;
#5032=EDGE_CURVE ( 'NONE', #20804, #14180, #1843, .T. ) ;
#5037=ORIENTED_EDGE ( 'NONE', *, *, #7234, .F. ) ;
#5038=AXIS2_PLACEMENT_3D ( 'NONE', #15547, #3562, #11445 ) ;
#5040=CARTESIAN_POINT ( 'NONE',  ( 46.81606138205705747, -33.21365173458013231, 70.96885009038120984 ) ) ;
#5046=PLANE ( 'NONE',  #25072 ) ;
#5052=LINE ( 'NONE', #8679, #1384 ) ;
#5089=ORIENTED_EDGE ( 'NONE', *, *, #23462, .T. ) ;
#5092=CYLINDRICAL_SURFACE ( 'NONE', #122, 1.500000000000000222 ) ;
#5109=( LENGTH_UNIT ( ) NAMED_UNIT ( * ) SI_UNIT ( .MILLI., .METRE. ) );
#5113=AXIS2_PLACEMENT_3D ( 'NONE', #24143, #22101, #8715 ) ;
#5123=STYLED_ITEM ( 'NONE', ( #1222 ), #11987 ) ;
#5127=PLANE ( 'NONE',  #21504 ) ;
#5135=CARTESIAN_POINT ( 'NONE',  ( 41.81606138205696510, -0.8482369431493732570, -3.067843137301039302 ) ) ;
#5136=ORIENTED_EDGE ( 'NONE', *, *, #23684, .F. ) ;
#5156=ORIENTED_EDGE ( 'NONE', *, *, #17368, .F. ) ;
#5158=DIRECTION ( 'NONE',  ( 1.000000000000000000, 3.469446951953611033E-15, 0.000000000000000000 ) ) ;
#5168=DIRECTION ( 'NONE',  ( -1.500536805400590970E-15, 0.6529557272876933549, 0.7573960774932753104 ) ) ;
#5182=VERTEX_POINT ( 'NONE', #6445 ) ;
#5183=CARTESIAN_POINT ( 'NONE',  ( 46.81606138205697221, -4.349482454670835274, -5.142398479549302515 ) ) ;
#5194=PLANE ( 'NONE',  #16779 ) ;
#5195=ORIENTED_EDGE ( 'NONE', *, *, #5617, .F. ) ;
#5213=EDGE_CURVE ( 'NONE', #8578, #20287, #14425, .T. ) ;
#5215=LINE ( 'NONE', #15000, #17896 ) ;
#5217=VERTEX_POINT ( 'NONE', #12250 ) ;
#5236=AXIS2_PLACEMENT_3D ( 'NONE', #15476, #11631, #13935 ) ;
#5238=VECTOR ( 'NONE', #15143, 1000.000000000000000 ) ;
#5239=CARTESIAN_POINT ( 'NONE',  ( 46.81606138205697221, -3.676927583119989684, -4.810479898036873259 ) ) ;
#5240=EDGE_CURVE ( 'NONE', #15010, #4631, #10312, .T. ) ;
#5253=VERTEX_POINT ( 'NONE', #14299 ) ;
#5262=DIRECTION ( 'NONE',  ( -1.000000000000000000, -2.999999999999999839E-15, 0.000000000000000000 ) ) ;
#5268=ORIENTED_EDGE ( 'NONE', *, *, #8278, .F. ) ;
#5273=VECTOR ( 'NONE', #10686, 1000.000000000000114 ) ;
#5275=CARTESIAN_POINT ( 'NONE',  ( 33.31606138205697931, -5.022037326221725273, -5.474317061061731771 ) ) ;
#5276=DIRECTION ( 'NONE',  ( 1.202852874072920494E-15, -0.3934158747763039088, 0.9193606199277819524 ) ) ;
#5279=CARTESIAN_POINT ( 'NONE',  ( 33.80827534892208064, -18.91453975041207158, 24.37026150481227305 ) ) ;
#5281=CARTESIAN_POINT ( 'NONE',  ( 29.81606138205707168, -37.26069504592558701, 64.48189387429259511 ) ) ;
#5285=FACE_OUTER_BOUND ( 'NONE', #9657, .T. ) ;
#5291=ORIENTED_EDGE ( 'NONE', *, *, #10192, .T. ) ;
#5306=AXIS2_PLACEMENT_3D ( 'NONE', #25146, #13581, #23351 ) ;
#5334=VERTEX_POINT ( 'NONE', #8009 ) ;
#5343=VERTEX_POINT ( 'NONE', #16603 ) ;
#5351=LINE ( 'NONE', #14626, #24140 ) ;
#5365=CARTESIAN_POINT ( 'NONE',  ( 31.56606138205697576, -5.022037326221730602, -5.474317061061731771 ) ) ;
#5377=CARTESIAN_POINT ( 'NONE',  ( 31.56606138205697576, -5.918777154956194053, -5.916875169744970187 ) ) ;
#5383=CARTESIAN_POINT ( 'NONE',  ( 46.81606138205695800, -0.2703287878657641974, 1.505452687840413972 ) ) ;
#5405=LINE ( 'NONE', #25473, #18747 ) ;
#5408=ORIENTED_EDGE ( 'NONE', *, *, #7068, .F. ) ;
#5409=FACE_BOUND ( 'NONE', #10337, .T. ) ;
#5429=VECTOR ( 'NONE', #23922, 1000.000000000000000 ) ;
#5460=FACE_OUTER_BOUND ( 'NONE', #3367, .T. ) ;
#5484=EDGE_CURVE ( 'NONE', #8869, #5253, #3072, .T. ) ;
#5486=ORIENTED_EDGE ( 'NONE', *, *, #3089, .F. ) ;
#5490=FACE_OUTER_BOUND ( 'NONE', #4456, .T. ) ;
#5493=AXIS2_PLACEMENT_3D ( 'NONE', #16908, #11248, #24604 ) ;
#5497=VERTEX_POINT ( 'NONE', #13009 ) ;
#5506=DIRECTION ( 'NONE',  ( 3.965082230804125881E-15, -0.8967398287344645613, -0.4425581086832361399 ) ) ;
#5514=ORIENTED_EDGE ( 'NONE', *, *, #14200, .F. ) ;
#5517=DIRECTION ( 'NONE',  ( -1.000000000000000000, -3.046270958365671426E-15, 5.272995181423179347E-17 ) ) ;
#5528=AXIS2_PLACEMENT_3D ( 'NONE', #10511, #18365, #2748 ) ;
#5539=CARTESIAN_POINT ( 'NONE',  ( 35.56606138205698642, -9.092667827980710271, 28.75914562266559926 ) ) ;
#5540=PRODUCT_DEFINITION_FORMATION_WITH_SPECIFIED_SOURCE ( 'ANY', '', #19167, .NOT_KNOWN. ) ;
#5556=CARTESIAN_POINT ( 'NONE',  ( 31.91606138205697363, -3.854803714928949798, -5.706129749257958572 ) ) ;
#5557=VECTOR ( 'NONE', #21244, 1000.000000000000000 ) ;
#5572=PLANE ( 'NONE',  #8965 ) ;
#5587=DIRECTION ( 'NONE',  ( -1.734723475976807292E-15, 0.7516416929448820339, 0.6595716529892350355 ) ) ;
#5588=DIRECTION ( 'NONE',  ( -2.048868001712896742E-15, 0.6595716529892345914, -0.7516416929448823669 ) ) ;
#5593=DIRECTION ( 'NONE',  ( 1.000000000000000000, 2.999999999999999839E-15, 0.000000000000000000 ) ) ;
#5617=EDGE_CURVE ( 'NONE', #9497, #4779, #2082, .T. ) ;
#5622=DIRECTION ( 'NONE',  ( -1.000000000000000000, -3.469446951953611033E-15, 0.000000000000000000 ) ) ;
#5633=LINE ( 'NONE', #17360, #8555 ) ;
#5643=ORIENTED_EDGE ( 'NONE', *, *, #7858, .F. ) ;
#5657=DIRECTION ( 'NONE',  ( -1.000000000000000000, -2.751104698760144965E-15, 1.228345504986737969E-16 ) ) ;
#5669=ORIENTED_EDGE ( 'NONE', *, *, #24235, .T. ) ;
#5690=DIRECTION ( 'NONE',  ( 1.000000000000000000, 3.388898908187273079E-15, 1.919289851541777660E-16 ) ) ;
#5691=ORIENTED_EDGE ( 'NONE', *, *, #5240, .T. ) ;
#5693=DIRECTION ( 'NONE',  ( 2.011972697750612571E-15, -0.6595716529892353686, 0.7516416929448815898 ) ) ;
#5710=DIRECTION ( 'NONE',  ( 1.327674326049719602E-15, -0.4425581086832399147, 0.8967398287344627850 ) ) ;
#5714=ORIENTED_EDGE ( 'NONE', *, *, #10317, .F. ) ;
#5727=CARTESIAN_POINT ( 'NONE',  ( 39.31606138205697931, -10.61256217995208040, 37.48782943861662886 ) ) ;
#5753=CARTESIAN_POINT ( 'NONE',  ( 46.81606138205706458, -34.55876147768182705, 70.30501292735635843 ) ) ;
#5758=AXIS2_PLACEMENT_3D ( 'NONE', #2370, #12448, #18237 ) ;
#5778=ORIENTED_EDGE ( 'NONE', *, *, #5032, .F. ) ;
#5784=LINE ( 'NONE', #19303, #5557 ) ;
#5803=VERTEX_POINT ( 'NONE', #4823 ) ;
#5824=EDGE_CURVE ( 'NONE', #20600, #5217, #2905, .T. ) ;
#5831=CARTESIAN_POINT ( 'NONE',  ( 36.06606138205695089, 2.967040633637572089, 4.322985289651505525 ) ) ;
#5836=ORIENTED_EDGE ( 'NONE', *, *, #24962, .T. ) ;
#5840=CARTESIAN_POINT ( 'NONE',  ( 36.31606138205702194, -20.48251210171517300, 31.50167136002490764 ) ) ;
#5850=ADVANCED_FACE ( 'NONE', ( #20415 ), #24392, .T. ) ;
#5858=ORIENTED_EDGE ( 'NONE', *, *, #8001, .F. ) ;
#5866=AXIS2_PLACEMENT_3D ( 'NONE', #4367, #2167, #4118 ) ;
#5867=LINE ( 'NONE', #12185, #11122 ) ;
#5868=LINE ( 'NONE', #3934, #5238 ) ;
#5871=FACE_OUTER_BOUND ( 'NONE', #10353, .T. ) ;
#5872=ORIENTED_EDGE ( 'NONE', *, *, #19057, .T. ) ;
#5874=CIRCLE ( 'NONE', #1320, 1.499999999999999778 ) ;
#5887=CIRCLE ( 'NONE', #25198, 1.750000000000001776 ) ;
#5888=CYLINDRICAL_SURFACE ( 'NONE', #12884, 0.7500000000000001110 ) ;
#5892=DIRECTION ( 'NONE',  ( -1.000000000000000000, -2.999999999999999839E-15, 0.000000000000000000 ) ) ;
#5898=PLANE ( 'NONE',  #6546 ) ;
#5905=ORIENTED_EDGE ( 'NONE', *, *, #12960, .T. ) ;
#5915=DIRECTION ( 'NONE',  ( 1.000000000000000000, 2.999999999999999839E-15, 0.000000000000000000 ) ) ;
#5920=LINE ( 'NONE', #3593, #914 ) ;
#5929=VERTEX_POINT ( 'NONE', #18742 ) ;
#5932=CARTESIAN_POINT ( 'NONE',  ( 38.31606138205696510, -3.195232061939692336, -6.457771442202879797 ) ) ;
#5943=ADVANCED_FACE ( 'NONE', ( #11398 ), #25017, .T. ) ;
#5944=ORIENTED_EDGE ( 'NONE', *, *, #16642, .T. ) ;
#5950=EDGE_CURVE ( 'NONE', #20277, #20897, #15252, .T. ) ;
#5952=LINE ( 'NONE', #23454, #18509 ) ;
#5954=CARTESIAN_POINT ( 'NONE',  ( 37.31606138205702194, -20.48251210171516590, 31.50167136002490764 ) ) ;
#5957=CARTESIAN_POINT ( 'NONE',  ( 30.81606138205697576, -4.349482454670884124, -5.142398479549302515 ) ) ;
#5958=ADVANCED_FACE ( 'NONE', ( #20931 ), #4958, .F. ) ;
#5975=ORIENTED_EDGE ( 'NONE', *, *, #12960, .F. ) ;
#5977=CARTESIAN_POINT ( 'NONE',  ( 38.31606138205696510, -1.965028424401967344, 1.888915691893686244 ) ) ;
#5984=VECTOR ( 'NONE', #6568, 1000.000000000000000 ) ;
#5985=ORIENTED_EDGE ( 'NONE', *, *, #3106, .F. ) ;
#5988=CARTESIAN_POINT ( 'NONE',  ( 46.81606138205697221, -4.349482454670835274, -5.142398479549302515 ) ) ;
#5989=EDGE_CURVE ( 'NONE', #23131, #10242, #24767, .T. ) ;
#6015=CARTESIAN_POINT ( 'NONE',  ( 46.81606138205705747, -32.32696853385078128, 75.83798663122490780 ) ) ;
#6030=EDGE_CURVE ( 'NONE', #16125, #20225, #5215, .T. ) ;
#6037=ORIENTED_EDGE ( 'NONE', *, *, #24840, .T. ) ;
#6041=FACE_OUTER_BOUND ( 'NONE', #21430, .T. ) ;
#6059=ORIENTED_EDGE ( 'NONE', *, *, #13143, .F. ) ;
#6069=ORIENTED_EDGE ( 'NONE', *, *, #9737, .T. ) ;
#6074=CARTESIAN_POINT ( 'NONE',  ( 36.31606138205700063, -13.36080775159014244, 37.40752645450730540 ) ) ;
#6075=DIRECTION ( 'NONE',  ( -1.000000000000000000, -2.999999999999999839E-15, 0.000000000000000000 ) ) ;
#6090=CARTESIAN_POINT ( 'NONE',  ( 46.81606138205701484, -19.40517585842700043, 23.66972737280834238 ) ) ;
#6099=DIRECTION ( 'NONE',  ( -1.000000000000000000, -3.469446951953611033E-15, 0.000000000000000000 ) ) ;
#6101=ADVANCED_FACE ( 'NONE', ( #15759 ), #4172, .T. ) ;
#6113=LINE ( 'NONE', #19900, #18630 ) ;
#6119=ORIENTED_EDGE ( 'NONE', *, *, #16404, .F. ) ;
#6133=ORIENTED_EDGE ( 'NONE', *, *, #23711, .T. ) ;
#6136=FACE_OUTER_BOUND ( 'NONE', #13133, .T. ) ;
#6143=ORIENTED_EDGE ( 'NONE', *, *, #15413, .T. ) ;
#6147=LINE ( 'NONE', #16180, #13301 ) ;
#6157=CARTESIAN_POINT ( 'NONE',  ( 44.71606138205695657, 0.5799492015812843793, -3.145019409304214530 ) ) ;
#6168=DIRECTION ( 'NONE',  ( -1.123589211228918605E-15, 0.4425581086832399147, -0.8967398287344627850 ) ) ;
#6176=EDGE_CURVE ( 'NONE', #1075, #12192, #15393, .T. ) ;
#6183=CARTESIAN_POINT ( 'NONE',  ( 36.31606138205698642, -8.139132291388525786, 32.47600601670134779 ) ) ;
#6187=LINE ( 'NONE', #3991, #25483 ) ;
#6193=CIRCLE ( 'NONE', #10736, 1.500000000000000222 ) ;
#6219=ORIENTED_EDGE ( 'NONE', *, *, #11381, .F. ) ;
#6238=FACE_OUTER_BOUND ( 'NONE', #17631, .T. ) ;
#6244=CARTESIAN_POINT ( 'NONE',  ( 41.81606138205697221, -3.103162021984027241, -5.046558096268735305 ) ) ;
#6255=EDGE_LOOP ( 'NONE', ( #17149, #780, #19183, #11557 ) ) ;
#6260=DIRECTION ( 'NONE',  ( -1.327674326049719602E-15, 0.4425581086832399147, -0.8967398287344627850 ) ) ;
#6275=CARTESIAN_POINT ( 'NONE',  ( 34.81606138205697221, -3.103162021984047669, -5.046558096268735305 ) ) ;
#6281=ADVANCED_FACE ( 'NONE', ( #10221 ), #17961, .F. ) ;
#6283=VECTOR ( 'NONE', #23805, 1000.000000000000000 ) ;
#6285=DIRECTION ( 'NONE',  ( 1.000000000000000000, 2.952017753711455077E-15, 9.722472704681867976E-17 ) ) ;
#6295=DIRECTION ( 'NONE',  ( 1.000000000000000000, 3.259265938791515726E-15, 1.279526567694519919E-16 ) ) ;
#6305=VECTOR ( 'NONE', #9192, 1000.000000000000000 ) ;
#6306=ORIENTED_EDGE ( 'NONE', *, *, #11386, .F. ) ;
#6308=CARTESIAN_POINT ( 'NONE',  ( 45.81606138205706458, -34.13844651005145181, 70.48338531520533934 ) ) ;
#6316=ORIENTED_EDGE ( 'NONE', *, *, #10381, .F. ) ;
#6326=VECTOR ( 'NONE', #10111, 1000.000000000000000 ) ;
#6339=LINE ( 'NONE', #2800, #7744 ) ;
#6344=DIRECTION ( 'NONE',  ( 1.000000000000000000, 2.870367030604242092E-15, -6.397632838472598363E-17 ) ) ;
#6347=LINE ( 'NONE', #6090, #22900 ) ;
#6352=ORIENTED_EDGE ( 'NONE', *, *, #6726, .T. ) ;
#6355=PLANE ( 'NONE',  #8657 ) ;
#6374=CARTESIAN_POINT ( 'NONE',  ( 44.71606138205697079, -3.195232061939673240, -6.457771442202879797 ) ) ;
#6375=ORIENTED_EDGE ( 'NONE', *, *, #9687, .T. ) ;
#6378=CARTESIAN_POINT ( 'NONE',  ( 46.81606138205701484, -19.40517585842700043, 23.66972737280834238 ) ) ;
#6391=DIRECTION ( 'NONE',  ( -1.000000000000000000, -3.965082230804126670E-15, 0.000000000000000000 ) ) ;
#6402=EDGE_LOOP ( 'NONE', ( #24125, #535, #17993, #5136 ) ) ;
#6445=CARTESIAN_POINT ( 'NONE',  ( 45.81606138205707168, -36.31746077171914067, 73.86860304758450013 ) ) ;
#6463=CYLINDRICAL_SURFACE ( 'NONE', #22590, 1.499999999999999778 ) ;
#6472=VERTEX_POINT ( 'NONE', #7368 ) ;
#6476=ORIENTED_EDGE ( 'NONE', *, *, #3571, .T. ) ;
#6487=ADVANCED_FACE ( 'NONE', ( #20512 ), #18831, .F. ) ;
#6488=AXIS2_PLACEMENT_3D ( 'NONE', #22704, #18977, #10746 ) ;
#6525=CIRCLE ( 'NONE', #2395, 4.000000000000000000 ) ;
#6527=VECTOR ( 'NONE', #2287, 1000.000000000000000 ) ;
#6529=DIRECTION ( 'NONE',  ( 1.327674326049701655E-15, -0.4425581086832336419, 0.8967398287344658936 ) ) ;
#6533=ORIENTED_EDGE ( 'NONE', *, *, #446, .F. ) ;
#6538=ORIENTED_EDGE ( 'NONE', *, *, #21591, .T. ) ;
#6540=DIRECTION ( 'NONE',  ( -1.000000000000000000, -3.091505625455828697E-15, -4.515976121274772923E-17 ) ) ;
#6546=AXIS2_PLACEMENT_3D ( 'NONE', #21991, #8088, #10272 ) ;
#6568=DIRECTION ( 'NONE',  ( 2.792262043613788535E-15, -0.8967398287344627850, -0.4425581086832399147 ) ) ;
#6573=LINE ( 'NONE', #21789, #9950 ) ;
#6587=DIRECTION ( 'NONE',  ( -2.048868001712896742E-15, 0.6595716529892345914, -0.7516416929448823669 ) ) ;
#6588=ADVANCED_FACE ( 'NONE', ( #9942, #1932 ), #9695, .T. ) ;
#6589=EDGE_LOOP ( 'NONE', ( #5486, #11021 ) ) ;
#6598=DIRECTION ( 'NONE',  ( 2.690219486203388234E-15, -0.8967398287344627850, -0.4425581086832399147 ) ) ;
#6601=ORIENTED_EDGE ( 'NONE', *, *, #16404, .T. ) ;
#6605=AXIS2_PLACEMENT_3D ( 'NONE', #20985, #1266, #9147 ) ;
#6616=AXIS2_PLACEMENT_3D ( 'NONE', #13484, #1736, #15794 ) ;
#6618=VECTOR ( 'NONE', #17352, 1000.000000000000000 ) ;
#6626=DIRECTION ( 'NONE',  ( -1.000000000000000000, -2.999999999999999839E-15, 0.000000000000000000 ) ) ;
#6640=ORIENTED_EDGE ( 'NONE', *, *, #8820, .T. ) ;
#6641=ORIENTED_EDGE ( 'NONE', *, *, #23106, .F. ) ;
#6644=CARTESIAN_POINT ( 'NONE',  ( 45.06606138205697221, -4.349482454670840603, -5.142398479549302515 ) ) ;
#6652=DIRECTION ( 'NONE',  ( 1.327674326049719602E-15, -0.4425581086832399147, 0.8967398287344627850 ) ) ;
#6653=EDGE_LOOP ( 'NONE', ( #13646, #1238, #15076, #290, #15202, #19941, #9352, #6533 ) ) ;
#6657=ADVANCED_FACE ( 'NONE', ( #3495 ), #3743, .F. ) ;
#6663=AXIS2_PLACEMENT_3D ( 'NONE', #5239, #11308, #9372 ) ;
#6669=CYLINDRICAL_SURFACE ( 'NONE', #21371, 1.500000000000000222 ) ;
#6672=DIRECTION ( 'NONE',  ( 1.000000000000000000, 3.469446951953611033E-15, 0.000000000000000000 ) ) ;
#6684=EDGE_LOOP ( 'NONE', ( #19081, #14327, #8974, #18448 ) ) ;
#6711=VECTOR ( 'NONE', #14707, 1000.000000000000000 ) ;
#6723=EDGE_CURVE ( 'NONE', #2101, #21215, #12010, .T. ) ;
#6724=CARTESIAN_POINT ( 'NONE',  ( 36.31606138205698642, -9.274586591516587930, 29.12776117315710067 ) ) ;
#6726=EDGE_CURVE ( 'NONE', #4631, #2880, #17930, .T. ) ;
#6739=VECTOR ( 'NONE', #1436, 1000.000000000000000 ) ;
#6741=LINE ( 'NONE', #9199, #25404 ) ;
#6743=ORIENTED_EDGE ( 'NONE', *, *, #13440, .F. ) ;
#6748=CARTESIAN_POINT ( 'NONE',  ( 35.91606138205694521, 3.586515973360777654, -0.5067327973472466329 ) ) ;
#6764=ORIENTED_EDGE ( 'NONE', *, *, #10589, .T. ) ;
#6784=ORIENTED_EDGE ( 'NONE', *, *, #3083, .F. ) ;
#6789=DIRECTION ( 'NONE',  ( 2.272188232479825545E-15, -0.7573960774932753104, 0.6529557272876933549 ) ) ;
#6790=ORIENTED_EDGE ( 'NONE', *, *, #22629, .F. ) ;
#6797=ORIENTED_EDGE ( 'NONE', *, *, #2623, .F. ) ;
#6808=LINE ( 'NONE', #3319, #9579 ) ;
#6829=DIRECTION ( 'NONE',  ( 0.000000000000000000, -0.7516416929448823669, -0.6595716529892345914 ) ) ;
#6856=CARTESIAN_POINT ( 'NONE',  ( 31.91606138205697363, -3.854803714928949798, -5.706129749257958572 ) ) ;
#6858=EDGE_CURVE ( 'NONE', #22022, #22279, #502, .T. ) ;
#6874=VERTEX_POINT ( 'NONE', #22411 ) ;
#6880=FACE_OUTER_BOUND ( 'NONE', #21998, .T. ) ;
#6885=DIRECTION ( 'NONE',  ( 0.000000000000000000, -0.7516416929448823669, -0.6595716529892345914 ) ) ;
#6895=ORIENTED_EDGE ( 'NONE', *, *, #23266, .T. ) ;
#6896=ORIENTED_EDGE ( 'NONE', *, *, #20605, .F. ) ;
#6897=EDGE_CURVE ( 'NONE', #9931, #2758, #1139, .T. ) ;
#6934=FACE_OUTER_BOUND ( 'NONE', #17279, .T. ) ;
#6954=CARTESIAN_POINT ( 'NONE',  ( 30.81606138205705037, -30.46100403034036219, 72.05704881431053366 ) ) ;
#6971=DIRECTION ( 'NONE',  ( 1.000000000000000000, 2.999999999999999839E-15, 0.000000000000000000 ) ) ;
#6980=DIRECTION ( 'NONE',  ( 1.000000000000000000, 2.751104698760144965E-15, -1.228345504986737969E-16 ) ) ;
#6989=PLANE ( 'NONE',  #7081 ) ;
#6995=DIRECTION ( 'NONE',  ( -1.327674326049721180E-15, 0.4425581086832404143, -0.8967398287344625629 ) ) ;
#7024=VERTEX_POINT ( 'NONE', #18799 ) ;
#7025=ORIENTED_EDGE ( 'NONE', *, *, #17415, .T. ) ;
#7029=EDGE_CURVE ( 'NONE', #21730, #17659, #5784, .T. ) ;
#7043=EDGE_CURVE ( 'NONE', #3839, #8686, #25283, .T. ) ;
#7052=EDGE_CURVE ( 'NONE', #4191, #20225, #23039, .T. ) ;
#7056=CARTESIAN_POINT ( 'NONE',  ( 41.06606138205698642, -9.092667827980692508, 28.75914562266559926 ) ) ;
#7059=EDGE_CURVE ( 'NONE', #180, #19523, #5405, .T. ) ;
#7068=EDGE_CURVE ( 'NONE', #5343, #1156, #13267, .T. ) ;
#7070=ORIENTED_EDGE ( 'NONE', *, *, #2786, .F. ) ;
#7081=AXIS2_PLACEMENT_3D ( 'NONE', #12926, #17805, #1809 ) ;
#7082=ORIENTED_EDGE ( 'NONE', *, *, #13045, .F. ) ;
#7083=VECTOR ( 'NONE', #6598, 1000.000000000000000 ) ;
#7084=CARTESIAN_POINT ( 'NONE',  ( 38.31606138205693668, 6.548188142891439689, 4.975198841308384523 ) ) ;
#7087=CARTESIAN_POINT ( 'NONE',  ( 44.71606138205692105, 12.25039015348823490, 8.426307875224583910 ) ) ;
#7092=CARTESIAN_POINT ( 'NONE',  ( 42.96606138205697789, -5.898435835062210586, -2.003809078978638247 ) ) ;
#7116=VECTOR ( 'NONE', #6168, 1000.000000000000000 ) ;
#7150=CARTESIAN_POINT ( 'NONE',  ( 31.91606138205695942, -0.07962245140798011878, -2.393377716359348817 ) ) ;
#7152=LINE ( 'NONE', #9474, #25441 ) ;
#7156=LINE ( 'NONE', #24645, #10615 ) ;
#7159=ORIENTED_EDGE ( 'NONE', *, *, #7292, .T. ) ;
#7160=CYLINDRICAL_SURFACE ( 'NONE', #9614, 1.000000000000000000 ) ;
#7164=CIRCLE ( 'NONE', #21132, 0.7500000000000006661 ) ;
#7165=SHAPE_REPRESENTATION_RELATIONSHIP ( 'NONE' , 'NONE' ,  #14735, #11987 ) ;
#7167=VECTOR ( 'NONE', #10831, 1000.000000000000114 ) ;
#7169=DIRECTION ( 'NONE',  ( 1.000000000000000000, 3.469446951953611033E-15, 0.000000000000000000 ) ) ;
#7184=CYLINDRICAL_SURFACE ( 'NONE', #1344, 4.000000000000000000 ) ;
#7203=ORIENTED_EDGE ( 'NONE', *, *, #12874, .T. ) ;
#7211=DIRECTION ( 'NONE',  ( -1.000000000000000000, -7.319250130266555251E-16, -4.595720054541213141E-15 ) ) ;
#7217=VECTOR ( 'NONE', #10948, 1000.000000000000114 ) ;
#7219=FACE_OUTER_BOUND ( 'NONE', #24893, .T. ) ;
#7225=ADVANCED_FACE ( 'NONE', ( #16201, #6041 ), #4617, .T. ) ;
#7228=EDGE_CURVE ( 'NONE', #15157, #4595, #2285, .T. ) ;
#7231=VERTEX_POINT ( 'NONE', #11985 ) ;
#7234=EDGE_CURVE ( 'NONE', #7231, #2274, #24055, .T. ) ;
#7239=LINE ( 'NONE', #5183, #24679 ) ;
#7248=CARTESIAN_POINT ( 'NONE',  ( 31.91606138205695942, 0.5799492015812461876, -3.145019409304214530 ) ) ;
#7250=DIRECTION ( 'NONE',  ( 1.327674326049719602E-15, -0.4425581086832399147, 0.8967398287344627850 ) ) ;
#7270=DIRECTION ( 'NONE',  ( -2.048868001712896742E-15, 0.6595716529892345914, -0.7516416929448823669 ) ) ;
#7271=CYLINDRICAL_SURFACE ( 'NONE', #19453, 3.000000000000000888 ) ;
#7282=ORIENTED_EDGE ( 'NONE', *, *, #4714, .F. ) ;
#7283=CIRCLE ( 'NONE', #13063, 4.000000000000000000 ) ;
#7284=AXIS2_PLACEMENT_3D ( 'NONE', #17821, #23468, #4024 ) ;
#7292=EDGE_CURVE ( 'NONE', #13994, #1644, #15945, .T. ) ;
#7294=FACE_OUTER_BOUND ( 'NONE', #2086, .T. ) ;
#7302=AXIS2_PLACEMENT_3D ( 'NONE', #8431, #24113, #16783 ) ;
#7308=CARTESIAN_POINT ( 'NONE',  ( 30.81606138205705037, -30.65246816789535345, 72.44500581826353880 ) ) ;
#7315=CARTESIAN_POINT ( 'NONE',  ( 42.96606138205698500, -6.570990706613058840, -2.335727660491067503 ) ) ;
#7321=CARTESIAN_POINT ( 'NONE',  ( 36.31606138205701484, -18.91453975041206093, 24.37026150481227305 ) ) ;
#7323=LINE ( 'NONE', #11712, #18495 ) ;
#7360=ORIENTED_EDGE ( 'NONE', *, *, #17415, .F. ) ;
#7367=ORIENTED_EDGE ( 'NONE', *, *, #15799, .T. ) ;
#7368=CARTESIAN_POINT ( 'NONE',  ( 33.66606138205698073, -6.230354416574667376, -1.331254207427787328 ) ) ;
#7376=AXIS2_PLACEMENT_3D ( 'NONE', #10360, #19640, #50 ) ;
#7381=AXIS2_PLACEMENT_3D ( 'NONE', #17259, #15188, #17521 ) ;
#7382=VERTEX_POINT ( 'NONE', #4742 ) ;
#7400=DIRECTION ( 'NONE',  ( 2.312964634635742267E-15, -0.8967398287344627850, -0.4425581086832398592 ) ) ;
#7403=VECTOR ( 'NONE', #22467, 1000.000000000000000 ) ;
#7404=ORIENTED_EDGE ( 'NONE', *, *, #7665, .T. ) ;
#7409=DIRECTION ( 'NONE',  ( 1.327674326049719602E-15, -0.4425581086832399147, 0.8967398287344627850 ) ) ;
#7411=VECTOR ( 'NONE', #17471, 1000.000000000000000 ) ;
#7420=CARTESIAN_POINT ( 'NONE',  ( 46.81606138205695089, 5.290470704224636833, -0.3848988112044732235 ) ) ;
#7422=CARTESIAN_POINT ( 'NONE',  ( 45.06606138205707879, -39.09901169483119077, 63.57464975149194686 ) ) ;
#7443=FACE_OUTER_BOUND ( 'NONE', #25009, .T. ) ;
#7445=DIRECTION ( 'NONE',  ( 0.000000000000000000, -0.7516416929448823669, -0.6595716529892345914 ) ) ;
#7454=CARTESIAN_POINT ( 'NONE',  ( 30.81606138205706813, -35.90867894478445521, 74.07034463014319670 ) ) ;
#7464=DIRECTION ( 'NONE',  ( -1.000000000000000000, -2.999999999999999839E-15, 0.000000000000000000 ) ) ;
#7471=CARTESIAN_POINT ( 'NONE',  ( 29.81606138205707168, -37.70325315460882365, 65.37863370302704880 ) ) ;
#7473=DIRECTION ( 'NONE',  ( 0.000000000000000000, 0.4425581086832400812, -0.8967398287344626739 ) ) ;
#7499=FACE_OUTER_BOUND ( 'NONE', #8229, .T. ) ;
#7507=ADVANCED_FACE ( 'NONE', ( #4863, #12991 ), #10927, .F. ) ;
#7513=EDGE_CURVE ( 'NONE', #1156, #13201, #84, .T. ) ;
#7516=LINE ( 'NONE', #13439, #18389 ) ;
#7527=ORIENTED_EDGE ( 'NONE', *, *, #8713, .F. ) ;
#7553=CYLINDRICAL_SURFACE ( 'NONE', #21266, 1.000000000000000888 ) ;
#7554=EDGE_CURVE ( 'NONE', #13632, #12758, #14496, .T. ) ;
#7560=ORIENTED_EDGE ( 'NONE', *, *, #10186, .F. ) ;
#7561=ORIENTED_EDGE ( 'NONE', *, *, #16350, .T. ) ;
#7572=CARTESIAN_POINT ( 'NONE',  ( 45.06606138205707879, -38.42645682328033985, 63.90656833300437256 ) ) ;
#7581=AXIS2_PLACEMENT_3D ( 'NONE', #2035, #5915, #9916 ) ;
#7589=DIRECTION ( 'NONE',  ( -1.000000000000000000, -2.751104698760144965E-15, 1.228345504986737969E-16 ) ) ;
#7603=LINE ( 'NONE', #5539, #9039 ) ;
#7614=DIRECTION ( 'NONE',  ( -1.000000000000000000, -3.046345864243081103E-15, -1.366653866685768465E-16 ) ) ;
#7616=CARTESIAN_POINT ( 'NONE',  ( 42.96606138205698500, -6.570990706613058840, -2.335727660491067503 ) ) ;
#7626=CARTESIAN_POINT ( 'NONE',  ( 36.31606138205702194, -20.30191568716149320, 23.22716926412510219 ) ) ;
#7628=DIRECTION ( 'NONE',  ( 1.000000000000000000, 2.999999999999999839E-15, 0.000000000000000000 ) ) ;
#7629=PLANE ( 'NONE',  #15355 ) ;
#7655=ORIENTED_EDGE ( 'NONE', *, *, #24182, .F. ) ;
#7665=EDGE_CURVE ( 'NONE', #11230, #20225, #3380, .T. ) ;
#7675=CARTESIAN_POINT ( 'NONE',  ( 42.96606138205698500, -7.345467396808729177, -0.7664329602057526891 ) ) ;
#7676=DIRECTION ( 'NONE',  ( -1.327674326049719602E-15, 0.4425581086832399147, -0.8967398287344627850 ) ) ;
#7686=VERTEX_POINT ( 'NONE', #23267 ) ;
#7702=CARTESIAN_POINT ( 'NONE',  ( 40.56606138205695089, 4.312150376739281477, 4.986822452676363149 ) ) ;
#7706=AXIS2_PLACEMENT_3D ( 'NONE', #24909, #7676, #21453 ) ;
#7711=DIRECTION ( 'NONE',  ( -2.048868001712899108E-15, 0.6595716529892353686, -0.7516416929448815898 ) ) ;
#7739=ORIENTED_EDGE ( 'NONE', *, *, #24012, .T. ) ;
#7744=VECTOR ( 'NONE', #22043, 1000.000000000000000 ) ;
#7752=EDGE_LOOP ( 'NONE', ( #7527, #17071, #12835, #19893 ) ) ;
#7756=CARTESIAN_POINT ( 'NONE',  ( 46.81606138205701484, -19.58709462196287632, 24.03834292329984379 ) ) ;
#7785=DIRECTION ( 'NONE',  ( 1.000000000000000000, 2.999999999999999839E-15, 0.000000000000000000 ) ) ;
#7788=AXIS2_PLACEMENT_3D ( 'NONE', #24063, #10427, #15705 ) ;
#7803=LINE ( 'NONE', #7675, #21797 ) ;
#7819=VERTEX_POINT ( 'NONE', #10137 ) ;
#7834=FACE_BOUND ( 'NONE', #23150, .T. ) ;
#7847=ADVANCED_FACE ( 'NONE', ( #24606 ), #6989, .T. ) ;
#7849=ORIENTED_EDGE ( 'NONE', *, *, #3407, .F. ) ;
#7854=DIRECTION ( 'NONE',  ( 1.123589211228918605E-15, -0.4425581086832399147, 0.8967398287344627850 ) ) ;
#7858=EDGE_CURVE ( 'NONE', #19743, #6874, #11501, .T. ) ;
#7912=DIRECTION ( 'NONE',  ( 0.000000000000000000, -0.4425581086832391930, 0.8967398287344632291 ) ) ;
#7921=EDGE_CURVE ( 'NONE', #24841, #22626, #13425, .T. ) ;
#7931=VERTEX_POINT ( 'NONE', #10076 ) ;
#7932=DIRECTION ( 'NONE',  ( -1.000000000000000000, -3.091505625455828697E-15, -4.515976121274772923E-17 ) ) ;
#7940=DIRECTION ( 'NONE',  ( 1.000000000000000000, 2.999999999999999839E-15, 0.000000000000000000 ) ) ;
#7957=LINE ( 'NONE', #2132, #19099 ) ;
#7963=AXIS2_PLACEMENT_3D ( 'NONE', #19879, #16374, #17956 ) ;
#7964=DIRECTION ( 'NONE',  ( -1.000000000000000000, -2.999999999999999839E-15, 0.000000000000000000 ) ) ;
#7969=AXIS2_PLACEMENT_3D ( 'NONE', #1704, #13707, #21685 ) ;
#7974=DIRECTION ( 'NONE',  ( 2.602085213965210642E-15, -0.8967398287344635621, -0.4425581086832386379 ) ) ;
#7979=EDGE_LOOP ( 'NONE', ( #10791, #19680, #7159, #2933 ) ) ;
#7992=ADVANCED_FACE ( 'NONE', ( #9946 ), #3747, .F. ) ;
#8001=EDGE_CURVE ( 'NONE', #19553, #7819, #5952, .T. ) ;
#8004=ORIENTED_EDGE ( 'NONE', *, *, #2002, .F. ) ;
#8009=CARTESIAN_POINT ( 'NONE',  ( 34.66606138205693810, 6.548188142891429919, 4.975198841308384523 ) ) ;
#8011=CARTESIAN_POINT ( 'NONE',  ( 46.81606138205695089, 5.290470704224636833, -0.3848988112044732235 ) ) ;
#8039=ORIENTED_EDGE ( 'NONE', *, *, #10589, .F. ) ;
#8057=LINE ( 'NONE', #6378, #16036 ) ;
#8071=EDGE_CURVE ( 'NONE', #18383, #4779, #22284, .T. ) ;
#8074=FACE_OUTER_BOUND ( 'NONE', #12506, .T. ) ;
#8080=FACE_OUTER_BOUND ( 'NONE', #19384, .T. ) ;
#8088=DIRECTION ( 'NONE',  ( -2.048868001712899108E-15, 0.6595716529892353686, -0.7516416929448815898 ) ) ;
#8089=CARTESIAN_POINT ( 'NONE',  ( 40.31606138205698642, -8.139132291388515128, 32.47600601670134779 ) ) ;
#8112=DIRECTION ( 'NONE',  ( -2.048868001712896742E-15, 0.6595716529892345914, -0.7516416929448823669 ) ) ;
#8116=FACE_OUTER_BOUND ( 'NONE', #8355, .T. ) ;
#8124=AXIS2_PLACEMENT_3D ( 'NONE', #3122, #19108, #24997 ) ;
#8134=DIRECTION ( 'NONE',  ( 1.327674326049719602E-15, -0.4425581086832399147, 0.8967398287344627850 ) ) ;
#8145=CARTESIAN_POINT ( 'NONE',  ( 46.81606138205707168, -36.31746077171913356, 73.86860304758450013 ) ) ;
#8148=DIRECTION ( 'NONE',  ( 1.000000000000000000, 2.999999999999999839E-15, 0.000000000000000000 ) ) ;
#8180=DIRECTION ( 'NONE',  ( -2.011972697750612571E-15, 0.6595716529892353686, -0.7516416929448815898 ) ) ;
#8185=DIRECTION ( 'NONE',  ( 0.000000000000000000, 0.6595716529892354796, -0.7516416929448814788 ) ) ;
#8191=AXIS2_PLACEMENT_3D ( 'NONE', #15192, #23295, #15574 ) ;
#8203=VERTEX_POINT ( 'NONE', #4273 ) ;
#8226=LINE ( 'NONE', #24165, #16523 ) ;
#8229=EDGE_LOOP ( 'NONE', ( #19877, #7367, #16833, #18895 ) ) ;
#8232=VECTOR ( 'NONE', #10753, 1000.000000000000000 ) ;
#8257=VERTEX_POINT ( 'NONE', #24956 ) ;
#8272=DIRECTION ( 'NONE',  ( -1.000000000000000000, -2.870367030604242092E-15, 6.397632838472598363E-17 ) ) ;
#8275=CARTESIAN_POINT ( 'NONE',  ( 40.56606138205695089, 4.754708485422523445, 4.090082623941899698 ) ) ;
#8277=CYLINDRICAL_SURFACE ( 'NONE', #7284, 1.749999999999999778 ) ;
#8278=EDGE_CURVE ( 'NONE', #5334, #18694, #24710, .T. ) ;
#8297=ADVANCED_FACE ( 'NONE', ( #7219 ), #9162, .F. ) ;
#8299=LINE ( 'NONE', #11921, #13740 ) ;
#8303=ADVANCED_FACE ( 'NONE', ( #14810, #5409, #882 ), #1409, .T. ) ;
#8323=ORIENTED_EDGE ( 'NONE', *, *, #16079, .T. ) ;
#8325=CARTESIAN_POINT ( 'NONE',  ( 46.81606138205707879, -39.09901169483115524, 63.57464975149190423 ) ) ;
#8331=CARTESIAN_POINT ( 'NONE',  ( 40.31606138205699352, -9.599063827782591929, 29.78523791026437095 ) ) ;
#8337=ORIENTED_EDGE ( 'NONE', *, *, #4215, .T. ) ;
#8338=LINE ( 'NONE', #23780, #17411 ) ;
#8341=CARTESIAN_POINT ( 'NONE',  ( 33.66606138205698073, -5.898435835062239008, -2.003809078978638247 ) ) ;
#8344=LINE ( 'NONE', #8089, #3217 ) ;
#8349=EDGE_CURVE ( 'NONE', #21215, #22719, #20528, .T. ) ;
#8352=ORIENTED_EDGE ( 'NONE', *, *, #18529, .T. ) ;
#8355=EDGE_LOOP ( 'NONE', ( #4592, #18766, #20672, #16551 ) ) ;
#8374=ORIENTED_EDGE ( 'NONE', *, *, #7554, .T. ) ;
#8378=ORIENTED_EDGE ( 'NONE', *, *, #3932, .T. ) ;
#8386=EDGE_CURVE ( 'NONE', #19553, #8450, #7603, .T. ) ;
#8391=CARTESIAN_POINT ( 'NONE',  ( 45.81606138205694378, 5.290470704224633280, -0.3848988112044732235 ) ) ;
#8409=CARTESIAN_POINT ( 'NONE',  ( 31.56606138205707879, -39.99575152356569419, 63.13209164280871022 ) ) ;
#8431=CARTESIAN_POINT ( 'NONE',  ( 33.80827534892208064, -20.02093502212017029, 26.61211107664843212 ) ) ;
#8450=VERTEX_POINT ( 'NONE', #3589 ) ;
#8458=CARTESIAN_POINT ( 'NONE',  ( 44.71606138205697079, -4.349482454670842380, -5.142398479549302515 ) ) ;
#8467=PLANE ( 'NONE',  #17815 ) ;
#8488=ADVANCED_FACE ( 'NONE', ( #22129 ), #16078, .F. ) ;
#8500=EDGE_CURVE ( 'NONE', #10242, #16874, #611, .T. ) ;
#8502=VERTEX_POINT ( 'NONE', #14031 ) ;
#8517=VECTOR ( 'NONE', #7250, 1000.000000000000000 ) ;
#8528=CARTESIAN_POINT ( 'NONE',  ( 41.81606138205696510, -1.975699482566714904, -4.057200616784870206 ) ) ;
#8551=CARTESIAN_POINT ( 'NONE',  ( 36.31606138205701484, -18.45164032183484792, 27.38658776684409091 ) ) ;
#8555=VECTOR ( 'NONE', #9268, 1000.000000000000000 ) ;
#8571=AXIS2_PLACEMENT_3D ( 'NONE', #4098, #19937, #10277 ) ;
#8572=CARTESIAN_POINT ( 'NONE',  ( 44.71606138205697789, -5.022037326221690634, -5.474317061061731771 ) ) ;
#8578=VERTEX_POINT ( 'NONE', #22260 ) ;
#8582=DIRECTION ( 'NONE',  ( 1.000000000000000000, 3.091505625455828697E-15, 4.515976121274772923E-17 ) ) ;
#8593=AXIS2_PLACEMENT_3D ( 'NONE', #9487, #15140, #7169 ) ;
#8597=LINE ( 'NONE', #16303, #308 ) ;
#8606=EDGE_LOOP ( 'NONE', ( #24099, #17694, #18517, #12315, #13266, #11306 ) ) ;
#8608=EDGE_CURVE ( 'NONE', #20703, #9852, #12115, .T. ) ;
#8614=CIRCLE ( 'NONE', #4903, 0.7499999999999985567 ) ;
#8623=ADVANCED_FACE ( 'NONE', ( #20339 ), #6669, .F. ) ;
#8624=EDGE_CURVE ( 'NONE', #20374, #13086, #12348, .T. ) ;
#8627=AXIS2_PLACEMENT_3D ( 'NONE', #10465, #10720, #18323 ) ;
#8631=ORIENTED_EDGE ( 'NONE', *, *, #20401, .T. ) ;
#8636=EDGE_CURVE ( 'NONE', #16929, #18597, #12744, .T. ) ;
#8647=AXIS2_PLACEMENT_3D ( 'NONE', #6074, #11629, #12014 ) ;
#8657=AXIS2_PLACEMENT_3D ( 'NONE', #14214, #16373, #12285 ) ;
#8663=ORIENTED_EDGE ( 'NONE', *, *, #4238, .T. ) ;
#8670=VERTEX_POINT ( 'NONE', #5135 ) ;
#8676=CARTESIAN_POINT ( 'NONE',  ( 40.31606138205701484, -18.45164032183483727, 27.38658776684409091 ) ) ;
#8679=CARTESIAN_POINT ( 'NONE',  ( 45.81606138205706458, -35.90867894478441968, 74.07034463014319670 ) ) ;
#8683=FACE_OUTER_BOUND ( 'NONE', #15037, .T. ) ;
#8684=EDGE_CURVE ( 'NONE', #21215, #7231, #4744, .T. ) ;
#8686=VERTEX_POINT ( 'NONE', #16979 ) ;
#8687=CARTESIAN_POINT ( 'NONE',  ( 33.66606138205694521, 5.651448314156965580, 4.532640732625139002 ) ) ;
#8688=DIRECTION ( 'NONE',  ( 1.327674326049709741E-15, -0.4425581086832367506, 0.8967398287344643393 ) ) ;
#8702=ORIENTED_EDGE ( 'NONE', *, *, #2002, .T. ) ;
#8711=ORIENTED_EDGE ( 'NONE', *, *, #14606, .T. ) ;
#8713=EDGE_CURVE ( 'NONE', #14019, #4191, #8745, .T. ) ;
#8715=DIRECTION ( 'NONE',  ( -3.965082230804125881E-15, 0.8967398287344645613, 0.4425581086832361399 ) ) ;
#8721=CARTESIAN_POINT ( 'NONE',  ( 40.31606138205701484, -18.91453975041205382, 24.37026150481227305 ) ) ;
#8723=ORIENTED_EDGE ( 'NONE', *, *, #16871, .T. ) ;
#8727=EDGE_CURVE ( 'NONE', #22626, #20600, #11050, .T. ) ;
#8728=FACE_OUTER_BOUND ( 'NONE', #1535, .T. ) ;
#8737=ORIENTED_EDGE ( 'NONE', *, *, #23711, .F. ) ;
#8745=LINE ( 'NONE', #10680, #4513 ) ;
#8748=DIRECTION ( 'NONE',  ( -1.271715504244016160E-15, 0.4425581086832399147, -0.8967398287344627850 ) ) ;
#8757=CARTESIAN_POINT ( 'NONE',  ( 42.96606138205697789, -5.898435835062210586, -2.003809078978638247 ) ) ;
#8766=EDGE_CURVE ( 'NONE', #13157, #7024, #12149, .T. ) ;
#8771=LINE ( 'NONE', #20742, #17882 ) ;
#8772=CIRCLE ( 'NONE', #7969, 1.000000000000012657 ) ;
#8786=CARTESIAN_POINT ( 'NONE',  ( 44.71606138205697079, -4.349482454670842380, -5.142398479549302515 ) ) ;
#8794=DIRECTION ( 'NONE',  ( -2.048868001712896742E-15, 0.6595716529892345914, -0.7516416929448823669 ) ) ;
#8799=FACE_OUTER_BOUND ( 'NONE', #12223, .T. ) ;
#8820=EDGE_CURVE ( 'NONE', #15268, #18307, #17044, .T. ) ;
#8824=VECTOR ( 'NONE', #10740, 1000.000000000000000 ) ;
#8825=CARTESIAN_POINT ( 'NONE',  ( 45.81606138205694378, 5.290470704224633280, -0.3848988112044732235 ) ) ;
#8828=ORIENTED_EDGE ( 'NONE', *, *, #3875, .T. ) ;
#8833=ORIENTED_EDGE ( 'NONE', *, *, #9299, .T. ) ;
#8846=VERTEX_POINT ( 'NONE', #6856 ) ;
#8850=DIRECTION ( 'NONE',  ( 0.000000000000000000, -0.4425581086832386379, 0.8967398287344635621 ) ) ;
#8854=CARTESIAN_POINT ( 'NONE',  ( 35.56606138205702194, -19.40517585842703596, 23.66972737280834238 ) ) ;
#8856=ADVANCED_FACE ( 'NONE', ( #13180 ), #10987, .T. ) ;
#8865=AXIS2_PLACEMENT_3D ( 'NONE', #3709, #17642, #1640 ) ;
#8869=VERTEX_POINT ( 'NONE', #16774 ) ;
#8874=DIRECTION ( 'NONE',  ( -1.327674326049719602E-15, 0.4425581086832399147, -0.8967398287344627850 ) ) ;
#8879=PLANE ( 'NONE',  #19226 ) ;
#8888=DIRECTION ( 'NONE',  ( -2.442401846778130416E-15, 0.8967398287344627850, 0.4425581086832399147 ) ) ;
#8894=CARTESIAN_POINT ( 'NONE',  ( 46.81606138205695089, 5.290470704224636833, -0.3848988112044732235 ) ) ;
#8896=ORIENTED_EDGE ( 'NONE', *, *, #22996, .T. ) ;
#8919=ORIENTED_EDGE ( 'NONE', *, *, #7554, .F. ) ;
#8940=AXIS2_PLACEMENT_3D ( 'NONE', #11254, #19106, #1442 ) ;
#8956=ORIENTED_EDGE ( 'NONE', *, *, #3932, .F. ) ;
#8957=DIRECTION ( 'NONE',  ( 2.792262043613788535E-15, -0.8967398287344627850, -0.4425581086832399147 ) ) ;
#8964=EDGE_CURVE ( 'NONE', #8502, #2101, #1923, .T. ) ;
#8965=AXIS2_PLACEMENT_3D ( 'NONE', #5957, #13312, #17424 ) ;
#8966=CARTESIAN_POINT ( 'NONE',  ( 34.66606138205693810, 6.105630034208187062, 5.871938670042847974 ) ) ;
#8973=EDGE_CURVE ( 'NONE', #13994, #2738, #15103, .T. ) ;
#8974=ORIENTED_EDGE ( 'NONE', *, *, #446, .T. ) ;
#8980=AXIS2_PLACEMENT_3D ( 'NONE', #22277, #20739, #3074 ) ;
#8983=AXIS2_PLACEMENT_3D ( 'NONE', #12045, #4310, #18213 ) ;
#8992=ORIENTED_EDGE ( 'NONE', *, *, #14928, .T. ) ;
#8998=DIRECTION ( 'NONE',  ( 1.000000000000000000, 2.602085213965208275E-15, 0.000000000000000000 ) ) ;
#9000=VECTOR ( 'NONE', #21230, 1000.000000000000000 ) ;
#9010=CARTESIAN_POINT ( 'NONE',  ( 42.96606138205698500, -7.345467396808729177, -0.7664329602057526891 ) ) ;
#9011=ORIENTED_EDGE ( 'NONE', *, *, #12683, .F. ) ;
#9025=ORIENTED_EDGE ( 'NONE', *, *, #24235, .F. ) ;
#9030=ADVANCED_FACE ( 'NONE', ( #7499 ), #21278, .F. ) ;
#9032=DIRECTION ( 'NONE',  ( 1.000000000000000000, 2.999999999999999839E-15, -5.603103565922885572E-33 ) ) ;
#9033=CARTESIAN_POINT ( 'NONE',  ( 34.81606138205696510, -1.975699482566735776, -4.057200616784870206 ) ) ;
#9039=VECTOR ( 'NONE', #23550, 1000.000000000000000 ) ;
#9041=DIRECTION ( 'NONE',  ( 0.000000000000000000, -0.4425581086832404143, 0.8967398287344625629 ) ) ;
#9050=AXIS2_PLACEMENT_3D ( 'NONE', #709, #1232, #18760 ) ;
#9057=ORIENTED_EDGE ( 'NONE', *, *, #9541, .F. ) ;
#9068=FACE_OUTER_BOUND ( 'NONE', #17879, .T. ) ;
#9072=CIRCLE ( 'NONE', #12364, 1.000000000000000000 ) ;
#9083=DIRECTION ( 'NONE',  ( -1.000000000000000000, -3.091505625455828697E-15, -4.515976121274772923E-17 ) ) ;
#9092=VERTEX_POINT ( 'NONE', #4649 ) ;
#9111=DIRECTION ( 'NONE',  ( 1.000000000000000000, 2.602085213965208275E-15, 0.000000000000000000 ) ) ;
#9113=ORIENTED_EDGE ( 'NONE', *, *, #18713, .T. ) ;
#9115=ADVANCED_FACE ( 'NONE', ( #2571 ), #22161, .T. ) ;
#9123=LINE ( 'NONE', #24797, #15626 ) ;
#9131=DIRECTION ( 'NONE',  ( -1.000000000000000000, -3.469446951953611033E-15, 0.000000000000000000 ) ) ;
#9134=CARTESIAN_POINT ( 'NONE',  ( 31.56606138205697576, -5.918777154956194053, -5.916875169744970187 ) ) ;
#9138=CARTESIAN_POINT ( 'NONE',  ( 46.81606138205697221, -6.425173154758061500, -4.890782882146171850 ) ) ;
#9147=DIRECTION ( 'NONE',  ( -1.000000000000000000, -2.999999999999999839E-15, 0.000000000000000000 ) ) ;
#9155=ORIENTED_EDGE ( 'NONE', *, *, #3571, .F. ) ;
#9162=CYLINDRICAL_SURFACE ( 'NONE', #3639, 0.7500000000000001110 ) ;
#9173=ORIENTED_EDGE ( 'NONE', *, *, #7292, .F. ) ;
#9185=ORIENTED_EDGE ( 'NONE', *, *, #3250, .F. ) ;
#9192=DIRECTION ( 'NONE',  ( 2.792262043613788535E-15, -0.8967398287344627850, -0.4425581086832399147 ) ) ;
#9199=CARTESIAN_POINT ( 'NONE',  ( 31.91606138205697718, -5.918777154956192277, -5.916875169744970187 ) ) ;
#9200=CIRCLE ( 'NONE', #2165, 1.000000000000000888 ) ;
#9201=ORIENTED_EDGE ( 'NONE', *, *, #3875, .F. ) ;
#9228=PLANE ( 'NONE',  #5306 ) ;
#9243=ORIENTED_EDGE ( 'NONE', *, *, #391, .T. ) ;
#9246=CARTESIAN_POINT ( 'NONE',  ( 41.06606138205703616, -23.83075694525941302, 32.63712566015296090 ) ) ;
#9266=ORIENTED_EDGE ( 'NONE', *, *, #21591, .F. ) ;
#9268=DIRECTION ( 'NONE',  ( 1.327674326049719602E-15, -0.4425581086832399147, 0.8967398287344627850 ) ) ;
#9278=CARTESIAN_POINT ( 'NONE',  ( 46.81606138205706458, -34.55876147768182705, 70.30501292735635843 ) ) ;
#9283=EDGE_CURVE ( 'NONE', #1959, #18383, #17137, .T. ) ;
#9286=CARTESIAN_POINT ( 'NONE',  ( 0.000000000000000000, 0.000000000000000000, 0.000000000000000000 ) ) ;
#9299=EDGE_CURVE ( 'NONE', #15655, #13108, #4897, .T. ) ;
#9319=LINE ( 'NONE', #13929, #23594 ) ;
#9352=ORIENTED_EDGE ( 'NONE', *, *, #2275, .F. ) ;
#9368=DIRECTION ( 'NONE',  ( 2.690219486203388234E-15, -0.8967398287344627850, -0.4425581086832399147 ) ) ;
#9371=STYLED_ITEM ( 'NONE', ( #15468 ), #322 ) ;
#9372=DIRECTION ( 'NONE',  ( -1.000000000000000000, -3.091505625455828697E-15, -4.515976121274772923E-17 ) ) ;
#9389=AXIS2_PLACEMENT_3D ( 'NONE', #24035, #7964, #13878 ) ;
#9419=DIRECTION ( 'NONE',  ( -1.000000000000000000, -2.999999999999999839E-15, 0.000000000000000000 ) ) ;
#9444=DIRECTION ( 'NONE',  ( 1.327674326049719602E-15, -0.4425581086832399147, 0.8967398287344627850 ) ) ;
#9450=VECTOR ( 'NONE', #20464, 1000.000000000000000 ) ;
#9462=EDGE_LOOP ( 'NONE', ( #15695, #20218, #2429, #1164 ) ) ;
#9465=FACE_OUTER_BOUND ( 'NONE', #2337, .T. ) ;
#9474=CARTESIAN_POINT ( 'NONE',  ( 46.81606138205707168, -35.90387122078352178, 69.64117576433150703 ) ) ;
#9487=CARTESIAN_POINT ( 'NONE',  ( 45.06606138205697221, -4.349482454670840603, -5.142398479549302515 ) ) ;
#9489=CARTESIAN_POINT ( 'NONE',  ( 44.71606138205697789, -5.022037326221690634, -5.474317061061731771 ) ) ;
#9497=VERTEX_POINT ( 'NONE', #3980 ) ;
#9516=DIRECTION ( 'NONE',  ( -1.327674326049719602E-15, 0.4425581086832399147, -0.8967398287344627850 ) ) ;
#9529=AXIS2_PLACEMENT_3D ( 'NONE', #21094, #15159, #5506 ) ;
#9539=CYLINDRICAL_SURFACE ( 'NONE', #25470, 1.000000000000014433 ) ;
#9541=EDGE_CURVE ( 'NONE', #20600, #11230, #5920, .T. ) ;
#9559=VECTOR ( 'NONE', #11206, 1000.000000000000000 ) ;
#9579=VECTOR ( 'NONE', #1118, 1000.000000000000114 ) ;
#9585=EDGE_CURVE ( 'NONE', #8846, #5343, #2974, .T. ) ;
#9601=DIRECTION ( 'NONE',  ( 2.690219486203388234E-15, -0.8967398287344627850, -0.4425581086832399147 ) ) ;
#9603=DIRECTION ( 'NONE',  ( -1.000000000000000000, -2.751104698760144965E-15, 1.228345504986737969E-16 ) ) ;
#9614=AXIS2_PLACEMENT_3D ( 'NONE', #18753, #16427, #8850 ) ;
#9621=LINE ( 'NONE', #5365, #7411 ) ;
#9645=DIRECTION ( 'NONE',  ( -1.327674326049719602E-15, 0.4425581086832399147, -0.8967398287344627850 ) ) ;
#9648=EDGE_CURVE ( 'NONE', #7819, #23131, #4621, .T. ) ;
#9657=EDGE_LOOP ( 'NONE', ( #5514, #9869, #14429, #15375 ) ) ;
#9687=EDGE_CURVE ( 'NONE', #2880, #16125, #22132, .T. ) ;
#9695=PLANE ( 'NONE',  #11330 ) ;
#9703=CARTESIAN_POINT ( 'NONE',  ( 40.56606138205695800, 0.3291273985901211896, 13.05748091128652533 ) ) ;
#9708=LINE ( 'NONE', #21550, #3259 ) ;
#9716=PLANE ( 'NONE',  #11661 ) ;
#9732=ORIENTED_EDGE ( 'NONE', *, *, #16090, .T. ) ;
#9737=EDGE_CURVE ( 'NONE', #13895, #19743, #24354, .T. ) ;
#9740=DIRECTION ( 'NONE',  ( -1.500536805400590970E-15, 0.6529557272876933549, 0.7573960774932753104 ) ) ;
#9750=CARTESIAN_POINT ( 'NONE',  ( 45.81606138205707168, -36.80651332587431313, 65.82119181171029254 ) ) ;
#9762=ORIENTED_EDGE ( 'NONE', *, *, #23489, .T. ) ;
#9765=DIRECTION ( 'NONE',  ( 2.690219486203388234E-15, -0.8967398287344627850, -0.4425581086832399147 ) ) ;
#9791=VECTOR ( 'NONE', #5693, 1000.000000000000114 ) ;
#9793=DIRECTION ( 'NONE',  ( -1.000000000000000000, -2.999999999999999839E-15, 0.000000000000000000 ) ) ;
#9800=PLANE ( 'NONE',  #10285 ) ;
#9804=ORIENTED_EDGE ( 'NONE', *, *, #14749, .F. ) ;
#9818=DIRECTION ( 'NONE',  ( -1.000000000000000000, -2.999999999999999839E-15, 0.000000000000000000 ) ) ;
#9831=LINE ( 'NONE', #5831, #16426 ) ;
#9833=CARTESIAN_POINT ( 'NONE',  ( 29.81606138205705037, -30.46100403034036219, 72.05704881431053366 ) ) ;
#9839=CARTESIAN_POINT ( 'NONE',  ( 45.81606138205707168, -37.26069504592553727, 64.48189387429259511 ) ) ;
#9852=VERTEX_POINT ( 'NONE', #15038 ) ;
#9854=EDGE_LOOP ( 'NONE', ( #1729, #1659, #23027, #3181 ) ) ;
#9861=EDGE_LOOP ( 'NONE', ( #23004, #8631, #10028, #20069 ) ) ;
#9869=ORIENTED_EDGE ( 'NONE', *, *, #22010, .F. ) ;
#9871=LINE ( 'NONE', #9750, #18822 ) ;
#9877=ORIENTED_EDGE ( 'NONE', *, *, #4883, .T. ) ;
#9881=CARTESIAN_POINT ( 'NONE',  ( 34.66606138205694521, 5.208890205473723611, 5.429380561359602453 ) ) ;
#9901=CARTESIAN_POINT ( 'NONE',  ( 31.56606138205697576, -5.918777154956194053, -5.916875169744970187 ) ) ;
#9911=VECTOR ( 'NONE', #8888, 1000.000000000000000 ) ;
#9916=DIRECTION ( 'NONE',  ( -3.469446951953572774E-15, 0.8967398287344627850, 0.4425581086832398037 ) ) ;
#9923=CYLINDRICAL_SURFACE ( 'NONE', #19693, 4.000000000000003553 ) ;
#9931=VERTEX_POINT ( 'NONE', #15676 ) ;
#9942=FACE_BOUND ( 'NONE', #19901, .T. ) ;
#9946=FACE_OUTER_BOUND ( 'NONE', #6255, .T. ) ;
#9950=VECTOR ( 'NONE', #23957, 1000.000000000000000 ) ;
#9952=CARTESIAN_POINT ( 'NONE',  ( 29.81606138205707168, -36.31746077171918330, 73.86860304758450013 ) ) ;
#9962=CARTESIAN_POINT ( 'NONE',  ( 43.31606138205697931, -6.570990706613057064, -2.335727660491067503 ) ) ;
#9968=LINE ( 'NONE', #23220, #22618 ) ;
#9987=VERTEX_POINT ( 'NONE', #17233 ) ;
#9996=ORIENTED_EDGE ( 'NONE', *, *, #9541, .T. ) ;
#10003=ORIENTED_EDGE ( 'NONE', *, *, #5950, .T. ) ;
#10005=ADVANCED_FACE ( 'NONE', ( #7443 ), #19040, .F. ) ;
#10012=AXIS2_PLACEMENT_3D ( 'NONE', #13249, #9516, #23273 ) ;
#10015=ORIENTED_EDGE ( 'NONE', *, *, #4238, .F. ) ;
#10028=ORIENTED_EDGE ( 'NONE', *, *, #11318, .T. ) ;
#10040=CIRCLE ( 'NONE', #23618, 0.7500000000000001110 ) ;
#10048=DIRECTION ( 'NONE',  ( 1.734723475976805517E-15, -0.4425581086832399702, 0.8967398287344627850 ) ) ;
#10049=EDGE_CURVE ( 'NONE', #18694, #7382, #18642, .T. ) ;
#10052=DIRECTION ( 'NONE',  ( 0.000000000000000000, -0.7516416929448823669, -0.6595716529892345914 ) ) ;
#10057=ORIENTED_EDGE ( 'NONE', *, *, #3250, .T. ) ;
#10060=DIRECTION ( 'NONE',  ( -1.225631768639319301E-15, 0.4425581086832399147, -0.8967398287344627850 ) ) ;
#10075=AXIS2_PLACEMENT_3D ( 'NONE', #17571, #9601, #6099 ) ;
#10076=CARTESIAN_POINT ( 'NONE',  ( 45.06606138205697931, -5.918777154956152309, -5.916875169744970187 ) ) ;
#10083=CARTESIAN_POINT ( 'NONE',  ( 45.81606138205705747, -33.21365173458013231, 70.96885009038120984 ) ) ;
#10094=ORIENTED_EDGE ( 'NONE', *, *, #3190, .F. ) ;
#10100=ORIENTED_EDGE ( 'NONE', *, *, #18080, .T. ) ;
#10111=DIRECTION ( 'NONE',  ( 2.792262043613788535E-15, -0.8967398287344627850, -0.4425581086832398592 ) ) ;
#10114=DIRECTION ( 'NONE',  ( -1.327674326049719602E-15, 0.4425581086832399147, -0.8967398287344627850 ) ) ;
#10117=LINE ( 'NONE', #16148, #10684 ) ;
#10125=CARTESIAN_POINT ( 'NONE',  ( 46.81606138205706458, -34.55876147768182705, 70.30501292735635843 ) ) ;
#10137=CARTESIAN_POINT ( 'NONE',  ( 35.56606138205703616, -23.83075694525942723, 32.63712566015296090 ) ) ;
#10139=ORIENTED_EDGE ( 'NONE', *, *, #11804, .T. ) ;
#10144=CARTESIAN_POINT ( 'NONE',  ( 43.31606138205697221, -3.118133360756952577, 16.65315793475036443 ) ) ;
#10176=ORIENTED_EDGE ( 'NONE', *, *, #11549, .T. ) ;
#10185=DIRECTION ( 'NONE',  ( -1.000000000000000000, -2.999999999999999839E-15, 0.000000000000000000 ) ) ;
#10186=EDGE_CURVE ( 'NONE', #13333, #5803, #8338, .T. ) ;
#10191=EDGE_CURVE ( 'NONE', #10854, #13157, #2514, .T. ) ;
#10192=EDGE_CURVE ( 'NONE', #7024, #5182, #6147, .T. ) ;
#10221=FACE_OUTER_BOUND ( 'NONE', #23883, .T. ) ;
#10242=VERTEX_POINT ( 'NONE', #23663 ) ;
#10246=VERTEX_POINT ( 'NONE', #6275 ) ;
#10248=CARTESIAN_POINT ( 'NONE',  ( 41.06606138205702194, -5.022037326221700404, -5.474317061061731771 ) ) ;
#10269=CARTESIAN_POINT ( 'NONE',  ( 41.06606138205702194, -20.30191568716147898, 23.22716926412510219 ) ) ;
#10272=DIRECTION ( 'NONE',  ( -1.000000000000000000, -3.243061817617045614E-15, -1.199556157213611407E-16 ) ) ;
#10277=DIRECTION ( 'NONE',  ( -1.133678928659556219E-16, 0.4425581086832399147, -0.8967398287344627850 ) ) ;
#10285=AXIS2_PLACEMENT_3D ( 'NONE', #15837, #7614, #21387 ) ;
#10312=LINE ( 'NONE', #4136, #20179 ) ;
#10317=EDGE_CURVE ( 'NONE', #13201, #20166, #20312, .T. ) ;
#10320=PLANE ( 'NONE',  #23113 ) ;
#10328=EDGE_CURVE ( 'NONE', #14345, #3268, #5887, .T. ) ;
#10337=EDGE_LOOP ( 'NONE', ( #5643, #15344, #23634, #23219, #24288, #5858, #19251, #298 ) ) ;
#10344=ORIENTED_EDGE ( 'NONE', *, *, #24091, .T. ) ;
#10353=EDGE_LOOP ( 'NONE', ( #4255, #1532, #9877, #23094 ) ) ;
#10355=CYLINDRICAL_SURFACE ( 'NONE', #7302, 0.7499999999999985567 ) ;
#10360=CARTESIAN_POINT ( 'NONE',  ( 29.81606138205707168, -36.80651332587436286, 65.82119181171029254 ) ) ;
#10361=VECTOR ( 'NONE', #9444, 1000.000000000000000 ) ;
#10362=ADVANCED_FACE ( 'NONE', ( #12593 ), #7160, .F. ) ;
#10369=DIRECTION ( 'NONE',  ( 2.312964634635742267E-15, -0.8967398287344634511, -0.4425581086832385824 ) ) ;
#10372=PLANE ( 'NONE',  #5758 ) ;
#10379=LINE ( 'NONE', #8325, #21092 ) ;
#10381=EDGE_CURVE ( 'NONE', #2880, #3879, #11672, .T. ) ;
#10401=AXIS2_PLACEMENT_3D ( 'NONE', #10144, #20183, #4474 ) ;
#10413=ORIENTED_EDGE ( 'NONE', *, *, #12874, .F. ) ;
#10422=CARTESIAN_POINT ( 'NONE',  ( 36.06606138205695800, 0.3291273985901090882, 13.05748091128652533 ) ) ;
#10427=DIRECTION ( 'NONE',  ( -1.327674326049719602E-15, 0.4425581086832399147, -0.8967398287344627850 ) ) ;
#10432=EDGE_LOOP ( 'NONE', ( #19077, #3134, #16598, #3305 ) ) ;
#10437=ORIENTED_EDGE ( 'NONE', *, *, #20498, .T. ) ;
#10465=CARTESIAN_POINT ( 'NONE',  ( 30.81606138205706102, -34.13844651005150155, 70.48338531520533934 ) ) ;
#10488=CARTESIAN_POINT ( 'NONE',  ( 36.31606138205699352, -10.61256217995208928, 37.48782943861662886 ) ) ;
#10490=CARTESIAN_POINT ( 'NONE',  ( 45.81606138205705037, -30.46100403034029114, 72.05704881431049103 ) ) ;
#10511=CARTESIAN_POINT ( 'NONE',  ( 31.56606138205707168, -38.42645682328038248, 63.90656833300437256 ) ) ;
#10525=ORIENTED_EDGE ( 'NONE', *, *, #7228, .F. ) ;
#10531=CARTESIAN_POINT ( 'NONE',  ( 36.31606138205702194, -20.48383445069737618, 23.59578481461660004 ) ) ;
#10544=ORIENTED_EDGE ( 'NONE', *, *, #594, .F. ) ;
#10545=DIRECTION ( 'NONE',  ( 1.000000000000000000, 2.751104698760144965E-15, -1.228345504986737969E-16 ) ) ;
#10550=CARTESIAN_POINT ( 'NONE',  ( 31.56606138205708589, -41.96692169274629691, 71.08048696288007307 ) ) ;
#10560=CARTESIAN_POINT ( 'NONE',  ( 46.81606138205706458, -34.54722833698617990, 70.28164373264664277 ) ) ;
#10568=DIRECTION ( 'NONE',  ( 0.000000000000000000, -0.7516416929448823669, -0.6595716529892345914 ) ) ;
#10582=DIRECTION ( 'NONE',  ( 1.000000000000000000, 2.999999999999999839E-15, 0.000000000000000000 ) ) ;
#10589=EDGE_CURVE ( 'NONE', #22719, #8502, #23111, .T. ) ;
#10601=CARTESIAN_POINT ( 'NONE',  ( 40.56606138205696510, -1.522470315718718270, 0.9921758631592225708 ) ) ;
#10614=EDGE_LOOP ( 'NONE', ( #8352, #17595, #15254, #20413, #8833, #8992 ) ) ;
#10615=VECTOR ( 'NONE', #11150, 1000.000000000000000 ) ;
#10632=DIRECTION ( 'NONE',  ( 1.000000000000000000, 2.751104698760144965E-15, -1.228345504986739201E-16 ) ) ;
#10646=DIRECTION ( 'NONE',  ( 2.048868001712898319E-15, -0.6595716529892350355, 0.7516416929448821449 ) ) ;
#10660=EDGE_CURVE ( 'NONE', #18307, #17722, #8299, .T. ) ;
#10664=ORIENTED_EDGE ( 'NONE', *, *, #18399, .F. ) ;
#10670=ORIENTED_EDGE ( 'NONE', *, *, #1368, .F. ) ;
#10672=LINE ( 'NONE', #2909, #17803 ) ;
#10680=CARTESIAN_POINT ( 'NONE',  ( 45.81606138205707168, -37.26069504592553727, 64.48189387429259511 ) ) ;
#10684=VECTOR ( 'NONE', #8180, 1000.000000000000114 ) ;
#10686=DIRECTION ( 'NONE',  ( 1.157642374584902751E-15, -0.3934158747763039088, 0.9193606199277819524 ) ) ;
#10688=VECTOR ( 'NONE', #22174, 1000.000000000000000 ) ;
#10690=ADVANCED_FACE ( 'NONE', ( #15890 ), #23748, .T. ) ;
#10703=CARTESIAN_POINT ( 'NONE',  ( 40.31606138205702194, -20.30191568716148254, 23.22716926412510219 ) ) ;
#10720=DIRECTION ( 'NONE',  ( 1.000000000000000000, 2.805550545906362824E-15, -9.596449257708899394E-17 ) ) ;
#10736=AXIS2_PLACEMENT_3D ( 'NONE', #9278, #3325, #18664 ) ;
#10740=DIRECTION ( 'NONE',  ( 2.690219486203388234E-15, -0.8967398287344627850, -0.4425581086832399147 ) ) ;
#10742=EDGE_CURVE ( 'NONE', #19743, #3268, #19895, .T. ) ;
#10743=ORIENTED_EDGE ( 'NONE', *, *, #12244, .T. ) ;
#10746=DIRECTION ( 'NONE',  ( -1.000000000000000000, -2.999999999999999839E-15, 0.000000000000000000 ) ) ;
#10751=CARTESIAN_POINT ( 'NONE',  ( 34.81606138205696510, -2.443590368994793760, -5.798199789213649424 ) ) ;
#10752=CIRCLE ( 'NONE', #14037, 1.500000000000000222 ) ;
#10753=DIRECTION ( 'NONE',  ( 2.792262043613788535E-15, -0.8967398287344627850, -0.4425581086832399147 ) ) ;
#10778=CARTESIAN_POINT ( 'NONE',  ( 46.81606138205705037, -30.46100403034029114, 72.05704881431049103 ) ) ;
#10783=AXIS2_PLACEMENT_3D ( 'NONE', #7572, #15286, #3687 ) ;
#10791=ORIENTED_EDGE ( 'NONE', *, *, #22807, .T. ) ;
#10803=CARTESIAN_POINT ( 'NONE',  ( 40.56606138205695800, 0.3291273985901211896, 13.05748091128652533 ) ) ;
#10806=DIRECTION ( 'NONE',  ( 2.782607932743246094E-15, -0.8967398287344627850, -0.4425581086832399147 ) ) ;
#10829=DIRECTION ( 'NONE',  ( -2.690219486203388234E-15, 0.8967398287344627850, 0.4425581086832399147 ) ) ;
#10831=DIRECTION ( 'NONE',  ( -2.515133600231165483E-15, 0.7516416929448815898, 0.6595716529892353686 ) ) ;
#10845=EDGE_CURVE ( 'NONE', #16878, #8203, #16781, .T. ) ;
#10846=VERTEX_POINT ( 'NONE', #8687 ) ;
#10854=VERTEX_POINT ( 'NONE', #10490 ) ;
#10904=DIRECTION ( 'NONE',  ( 0.000000000000000000, 0.8967398287344627850, 0.4425581086832398037 ) ) ;
#10921=ORIENTED_EDGE ( 'NONE', *, *, #18708, .F. ) ;
#10922=ORIENTED_EDGE ( 'NONE', *, *, #8766, .F. ) ;
#10923=CARTESIAN_POINT ( 'NONE',  ( 29.81606138205696155, -0.2703287878658162113, 1.505452687840413972 ) ) ;
#10927=PLANE ( 'NONE',  #23138 ) ;
#10937=DIRECTION ( 'NONE',  ( -1.000000000000000000, -3.087130386257447501E-15, -3.221081844416023957E-17 ) ) ;
#10942=ORIENTED_EDGE ( 'NONE', *, *, #14483, .F. ) ;
#10948=DIRECTION ( 'NONE',  ( 1.202852874072920494E-15, -0.3934158747763039088, 0.9193606199277819524 ) ) ;
#10978=CARTESIAN_POINT ( 'NONE',  ( 30.81606138205706813, -36.31746077171918330, 73.86860304758450013 ) ) ;
#10987=CYLINDRICAL_SURFACE ( 'NONE', #16648, 3.999999999999999556 ) ;
#10993=CIRCLE ( 'NONE', #14279, 4.000000000000000000 ) ;
#10998=VECTOR ( 'NONE', #20630, 1000.000000000000000 ) ;
#11013=LINE ( 'NONE', #20932, #23148 ) ;
#11015=DIRECTION ( 'NONE',  ( 1.000000000000000000, 2.999999999999999839E-15, 0.000000000000000000 ) ) ;
#11020=DIRECTION ( 'NONE',  ( -2.254925078834644814E-15, 0.7516416929448815898, 0.6595716529892353686 ) ) ;
#11021=ORIENTED_EDGE ( 'NONE', *, *, #1667, .F. ) ;
#11029=LINE ( 'NONE', #14761, #4475 ) ;
#11033=CARTESIAN_POINT ( 'NONE',  ( 43.31606138205700063, -14.32738121993773994, 11.12118157620986558 ) ) ;
#11038=ORIENTED_EDGE ( 'NONE', *, *, #14749, .T. ) ;
#11050=LINE ( 'NONE', #9134, #23221 ) ;
#11057=DIRECTION ( 'NONE',  ( 2.602085213965210642E-15, -0.8967398287344635621, -0.4425581086832386379 ) ) ;
#11063=DIRECTION ( 'NONE',  ( -1.327674326049719602E-15, 0.4425581086832399147, -0.8967398287344627850 ) ) ;
#11068=ORIENTED_EDGE ( 'NONE', *, *, #15109, .T. ) ;
#11077=VECTOR ( 'NONE', #4122, 1000.000000000000000 ) ;
#11096=CARTESIAN_POINT ( 'NONE',  ( 40.56606138205695089, 4.754708485422523445, 4.090082623941899698 ) ) ;
#11120=CARTESIAN_POINT ( 'NONE',  ( 30.81606138205707168, -36.80651332587435576, 65.82119181171029254 ) ) ;
#11122=VECTOR ( 'NONE', #20024, 1000.000000000000000 ) ;
#11133=VECTOR ( 'NONE', #13669, 1000.000000000000000 ) ;
#11143=ORIENTED_EDGE ( 'NONE', *, *, #16871, .F. ) ;
#11150=DIRECTION ( 'NONE',  ( -1.000000000000000000, -3.046270958365671426E-15, 5.272995181423179347E-17 ) ) ;
#11159=EDGE_CURVE ( 'NONE', #16874, #8450, #23931, .T. ) ;
#11168=DIRECTION ( 'NONE',  ( 1.000000000000000000, 2.999999999999999839E-15, 0.000000000000000000 ) ) ;
#11180=EDGE_LOOP ( 'NONE', ( #20920, #4033, #15905, #6316 ) ) ;
#11185=VECTOR ( 'NONE', #13617, 1000.000000000000000 ) ;
#11206=DIRECTION ( 'NONE',  ( -2.792262043613788535E-15, 0.8967398287344627850, 0.4425581086832398592 ) ) ;
#11230=VERTEX_POINT ( 'NONE', #18035 ) ;
#11247=CARTESIAN_POINT ( 'NONE',  ( 46.81606138205705037, -30.46100403034031245, 72.05704881431053366 ) ) ;
#11248=DIRECTION ( 'NONE',  ( -1.000000000000000000, -2.999999999999999839E-15, 0.000000000000000000 ) ) ;
#11254=CARTESIAN_POINT ( 'NONE',  ( 31.91606138205697363, -4.349482454670880571, -5.142398479549302515 ) ) ;
#11255=CIRCLE ( 'NONE', #4262, 1.750000000000001554 ) ;
#11259=ADVANCED_FACE ( 'NONE', ( #6934 ), #18656, .F. ) ;
#11276=AXIS2_PLACEMENT_3D ( 'NONE', #14950, #9419, #13153 ) ;
#11277=DIRECTION ( 'NONE',  ( 0.000000000000000000, -0.7516416929448823669, -0.6595716529892345914 ) ) ;
#11306=ORIENTED_EDGE ( 'NONE', *, *, #11772, .T. ) ;
#11308=DIRECTION ( 'NONE',  ( -2.792262043613788535E-15, 0.8967398287344627850, 0.4425581086832399147 ) ) ;
#11313=ORIENTED_EDGE ( 'NONE', *, *, #2038, .T. ) ;
#11316=CARTESIAN_POINT ( 'NONE',  ( 46.81606138205701484, -19.68901644060769485, 25.93955620509757409 ) ) ;
#11318=EDGE_CURVE ( 'NONE', #17659, #15674, #21904, .T. ) ;
#11330=AXIS2_PLACEMENT_3D ( 'NONE', #19591, #23581, #3 ) ;
#11348=DIRECTION ( 'NONE',  ( -1.000000000000000000, -2.999999999999999839E-15, 0.000000000000000000 ) ) ;
#11381=EDGE_CURVE ( 'NONE', #2625, #21683, #14788, .T. ) ;
#11386=EDGE_CURVE ( 'NONE', #12298, #9987, #6808, .T. ) ;
#11398=FACE_OUTER_BOUND ( 'NONE', #23903, .T. ) ;
#11402=FACE_BOUND ( 'NONE', #17929, .T. ) ;
#11414=DIRECTION ( 'NONE',  ( 1.327674326049721180E-15, -0.4425581086832404143, 0.8967398287344625629 ) ) ;
#11417=DIRECTION ( 'NONE',  ( -2.048868001712899108E-15, 0.6595716529892353686, -0.7516416929448815898 ) ) ;
#11418=DIRECTION ( 'NONE',  ( -1.327674326049719602E-15, 0.4425581086832399147, -0.8967398287344627850 ) ) ;
#11421=FACE_OUTER_BOUND ( 'NONE', #14822, .T. ) ;
#11433=DIRECTION ( 'NONE',  ( -1.000000000000000000, -2.976348234363322057E-15, -2.784991061251119320E-16 ) ) ;
#11434=ORIENTED_EDGE ( 'NONE', *, *, #1072, .T. ) ;
#11435=CYLINDRICAL_SURFACE ( 'NONE', #16085, 1.750000000000000222 ) ;
#11443=VECTOR ( 'NONE', #24449, 1000.000000000000000 ) ;
#11445=DIRECTION ( 'NONE',  ( 0.000000000000000000, 0.4425581086832400812, -0.8967398287344626739 ) ) ;
#11460=EDGE_CURVE ( 'NONE', #18144, #12687, #12460, .T. ) ;
#11465=ORIENTED_EDGE ( 'NONE', *, *, #15511, .T. ) ;
#11473=EDGE_CURVE ( 'NONE', #17369, #23160, #5874, .T. ) ;
#11484=DIRECTION ( 'NONE',  ( -2.412663730047099099E-15, 0.8967398287344627850, 0.4425581086832399147 ) ) ;
#11501=LINE ( 'NONE', #7756, #24749 ) ;
#11505=EDGE_CURVE ( 'NONE', #21683, #18450, #25190, .T. ) ;
#11513=VECTOR ( 'NONE', #18140, 1000.000000000000000 ) ;
#11528=EDGE_LOOP ( 'NONE', ( #1695, #5975, #23522, #24804 ) ) ;
#11539=EDGE_LOOP ( 'NONE', ( #6743, #16066, #5291, #9732 ) ) ;
#11542=ORIENTED_EDGE ( 'NONE', *, *, #4498, .T. ) ;
#11546=ORIENTED_EDGE ( 'NONE', *, *, #15413, .F. ) ;
#11549=EDGE_CURVE ( 'NONE', #23228, #17369, #19164, .T. ) ;
#11557=ORIENTED_EDGE ( 'NONE', *, *, #22629, .T. ) ;
#11561=ORIENTED_EDGE ( 'NONE', *, *, #22452, .F. ) ;
#11586=VERTEX_POINT ( 'NONE', #7702 ) ;
#11597=FACE_OUTER_BOUND ( 'NONE', #9861, .T. ) ;
#11601=ADVANCED_FACE ( 'NONE', ( #2268 ), #12211, .F. ) ;
#11607=DIRECTION ( 'NONE',  ( 0.000000000000000000, -0.7516416929448823669, -0.6595716529892345914 ) ) ;
#11629=DIRECTION ( 'NONE',  ( 1.000000000000000000, 3.001186103030333510E-15, 2.281710121244060993E-16 ) ) ;
#11631=DIRECTION ( 'NONE',  ( -2.690219486203388234E-15, 0.8967398287344627850, 0.4425581086832399147 ) ) ;
#11633=ORIENTED_EDGE ( 'NONE', *, *, #19801, .F. ) ;
#11639=AXIS2_PLACEMENT_3D ( 'NONE', #2919, #22771, #11057 ) ;
#11649=EDGE_LOOP ( 'NONE', ( #9057, #23184, #238, #24077, #8956, #20542 ) ) ;
#11661=AXIS2_PLACEMENT_3D ( 'NONE', #13823, #26, #13574 ) ;
#11669=EDGE_LOOP ( 'NONE', ( #22852, #10743, #5714, #24761 ) ) ;
#11672=CIRCLE ( 'NONE', #20280, 0.7500000000000006661 ) ;
#11680=CYLINDRICAL_SURFACE ( 'NONE', #24534, 4.000000000000003553 ) ;
#11686=ORIENTED_EDGE ( 'NONE', *, *, #4866, .T. ) ;
#11697=ORIENTED_EDGE ( 'NONE', *, *, #20830, .F. ) ;
#11704=ORIENTED_EDGE ( 'NONE', *, *, #24021, .F. ) ;
#11711=ADVANCED_FACE ( 'NONE', ( #16057 ), #8467, .T. ) ;
#11712=CARTESIAN_POINT ( 'NONE',  ( 46.81606138205700063, -13.43064139120326672, 11.56373968489310755 ) ) ;
#11718=ORIENTED_EDGE ( 'NONE', *, *, #15530, .T. ) ;
#11736=AXIS2_PLACEMENT_3D ( 'NONE', #11247, #2844, #1170 ) ;
#11760=DIRECTION ( 'NONE',  ( 1.067465804653198538E-15, -0.4425581086832399147, 0.8967398287344627850 ) ) ;
#11763=DIRECTION ( 'NONE',  ( -2.690219486203388234E-15, 0.8967398287344627850, 0.4425581086832399147 ) ) ;
#11772=EDGE_CURVE ( 'NONE', #10846, #5334, #9200, .T. ) ;
#11802=CARTESIAN_POINT ( 'NONE',  ( 42.96606138205698500, -6.570990706613058840, -2.335727660491067503 ) ) ;
#11804=EDGE_CURVE ( 'NONE', #9092, #10854, #834, .T. ) ;
#11829=DIRECTION ( 'NONE',  ( 2.690219486203388234E-15, -0.8967398287344627850, -0.4425581086832399147 ) ) ;
#11845=ORIENTED_EDGE ( 'NONE', *, *, #5213, .F. ) ;
#11852=COLOUR_RGB ( '', 0.09019608, 0.27058824, 0.51372549) ;
#11872=ORIENTED_EDGE ( 'NONE', *, *, #5014, .T. ) ;
#11903=CARTESIAN_POINT ( 'NONE',  ( 40.71606138205696368, 0.5799492015812739432, -3.145019409304214530 ) ) ;
#11904=CARTESIAN_POINT ( 'NONE',  ( 36.31606138205702194, -20.30191568716149320, 23.22716926412510219 ) ) ;
#11907=ORIENTED_EDGE ( 'NONE', *, *, #24135, .T. ) ;
#11921=CARTESIAN_POINT ( 'NONE',  ( 31.91606138205697363, -3.929900956088018038, -7.102449327239662935 ) ) ;
#11927=ORIENTED_EDGE ( 'NONE', *, *, #14894, .F. ) ;
#11959=ADVANCED_FACE ( 'NONE', ( #21317 ), #24905, .F. ) ;
#11960=ORIENTED_EDGE ( 'NONE', *, *, #23090, .F. ) ;
#11962=VECTOR ( 'NONE', #3491, 1000.000000000000114 ) ;
#11966=VECTOR ( 'NONE', #427, 1000.000000000000000 ) ;
#11972=LINE ( 'NONE', #2523, #14316 ) ;
#11985=CARTESIAN_POINT ( 'NONE',  ( 40.31606138205701484, -19.34838015056930161, 26.94402965816085072 ) ) ;
#11987=ADVANCED_BREP_SHAPE_REPRESENTATION ( '', ( #322, #2000 ), #3041 ) ;
#11999=DIRECTION ( 'NONE',  ( -1.000000000000000000, -3.046270958365671426E-15, 5.272995181423179347E-17 ) ) ;
#12001=ORIENTED_EDGE ( 'NONE', *, *, #24012, .F. ) ;
#12008=( NAMED_UNIT ( * ) PLANE_ANGLE_UNIT ( ) SI_UNIT ( $, .RADIAN. ) );
#12009=ORIENTED_EDGE ( 'NONE', *, *, #12027, .T. ) ;
#12010=LINE ( 'NONE', #23826, #5984 ) ;
#12014=DIRECTION ( 'NONE',  ( -1.123589211228918605E-15, 0.4425581086832399147, -0.8967398287344627850 ) ) ;
#12026=CIRCLE ( 'NONE', #20230, 3.000000000000000888 ) ;
#12027=EDGE_CURVE ( 'NONE', #9092, #18170, #1594, .T. ) ;
#12045=CARTESIAN_POINT ( 'NONE',  ( 45.81606138205706458, -34.55876147768182705, 70.30501292735635843 ) ) ;
#12070=ORIENTED_EDGE ( 'NONE', *, *, #13143, .T. ) ;
#12089=CARTESIAN_POINT ( 'NONE',  ( 36.31606138205699352, -10.17000407126884731, 36.59108960988216808 ) ) ;
#12092=CARTESIAN_POINT ( 'NONE',  ( 46.81606138205706458, -34.55876147768182705, 70.30501292735635843 ) ) ;
#12108=CIRCLE ( 'NONE', #3444, 1.499999999999999778 ) ;
#12111=VECTOR ( 'NONE', #5276, 1000.000000000000114 ) ;
#12115=LINE ( 'NONE', #10422, #2436 ) ;
#12149=CIRCLE ( 'NONE', #13376, 3.999999999999997335 ) ;
#12161=ORIENTED_EDGE ( 'NONE', *, *, #3486, .T. ) ;
#12168=ORIENTED_EDGE ( 'NONE', *, *, #15206, .F. ) ;
#12175=VECTOR ( 'NONE', #1897, 1000.000000000000000 ) ;
#12185=CARTESIAN_POINT ( 'NONE',  ( 40.31606138205699352, -9.092667827980694284, 28.75914562266559926 ) ) ;
#12189=EDGE_CURVE ( 'NONE', #16878, #8257, #6113, .T. ) ;
#12192=VERTEX_POINT ( 'NONE', #6374 ) ;
#12193=CARTESIAN_POINT ( 'NONE',  ( 46.81606138205707168, -37.26069504592553017, 64.48189387429259511 ) ) ;
#12198=VERTEX_POINT ( 'NONE', #16018 ) ;
#12205=ORIENTED_EDGE ( 'NONE', *, *, #14928, .F. ) ;
#12211=PLANE ( 'NONE',  #10401 ) ;
#12223=EDGE_LOOP ( 'NONE', ( #21441, #18254, #15758, #18829 ) ) ;
#12226=CARTESIAN_POINT ( 'NONE',  ( 38.31606138205695089, 2.967040633637578750, 4.322985289651505525 ) ) ;
#12238=DIRECTION ( 'NONE',  ( -1.000000000000000000, -3.091505625455828697E-15, -4.515976121274771690E-17 ) ) ;
#12244=EDGE_CURVE ( 'NONE', #22626, #20166, #11255, .T. ) ;
#12250=CARTESIAN_POINT ( 'NONE',  ( 29.81606138205707879, -38.42645682328038959, 63.90656833300437256 ) ) ;
#12260=CARTESIAN_POINT ( 'NONE',  ( 30.81606138205707879, -39.99575152356569419, 63.13209164280871022 ) ) ;
#12261=FACE_BOUND ( 'NONE', #23951, .T. ) ;
#12271=AXIS2_PLACEMENT_3D ( 'NONE', #19808, #14015, #2144 ) ;
#12285=DIRECTION ( 'NONE',  ( -1.000000000000000000, -2.999999999999999839E-15, 0.000000000000000000 ) ) ;
#12294=VECTOR ( 'NONE', #4220, 1000.000000000000000 ) ;
#12298=VERTEX_POINT ( 'NONE', #6748 ) ;
#12305=DIRECTION ( 'NONE',  ( 1.000000000000000000, 2.973811673103095397E-15, 0.000000000000000000 ) ) ;
#12311=ORIENTED_EDGE ( 'NONE', *, *, #22807, .F. ) ;
#12315=ORIENTED_EDGE ( 'NONE', *, *, #15530, .F. ) ;
#12316=CARTESIAN_POINT ( 'NONE',  ( 33.66606138205698073, -5.898435835062239008, -2.003809078978638247 ) ) ;
#12342=VECTOR ( 'NONE', #1411, 1000.000000000000000 ) ;
#12348=CIRCLE ( 'NONE', #22607, 1.000000000000000888 ) ;
#12361=AXIS2_PLACEMENT_3D ( 'NONE', #19121, #18861, #7400 ) ;
#12364=AXIS2_PLACEMENT_3D ( 'NONE', #12509, #4630, #4505 ) ;
#12366=CARTESIAN_POINT ( 'NONE',  ( 45.81606138205697221, -4.349482454670838827, -5.142398479549302515 ) ) ;
#12369=( NAMED_UNIT ( * ) PLANE_ANGLE_UNIT ( ) SI_UNIT ( $, .RADIAN. ) );
#12377=PLANE ( 'NONE',  #13601 ) ;
#12380=VECTOR ( 'NONE', #7711, 1000.000000000000114 ) ;
#12394=VECTOR ( 'NONE', #14803, 1000.000000000000000 ) ;
#12431=ORIENTED_EDGE ( 'NONE', *, *, #12633, .F. ) ;
#12432=CARTESIAN_POINT ( 'NONE',  ( 29.81606138205707168, -36.80651332587436286, 65.82119181171029254 ) ) ;
#12444=ORIENTED_EDGE ( 'NONE', *, *, #14126, .T. ) ;
#12446=ORIENTED_EDGE ( 'NONE', *, *, #16170, .F. ) ;
#12448=DIRECTION ( 'NONE',  ( -1.327674326049719602E-15, 0.4425581086832399147, -0.8967398287344627850 ) ) ;
#12452=ORIENTED_EDGE ( 'NONE', *, *, #11505, .T. ) ;
#12455=CARTESIAN_POINT ( 'NONE',  ( 41.81606138205696510, -0.8482369431493732570, -3.067843137301039302 ) ) ;
#12460=CIRCLE ( 'NONE', #5038, 1.750000000000000222 ) ;
#12461=DIRECTION ( 'NONE',  ( -1.000000000000000000, -3.046345864243081103E-15, -1.366653866685768465E-16 ) ) ;
#12503=VECTOR ( 'NONE', #6995, 1000.000000000000000 ) ;
#12506=EDGE_LOOP ( 'NONE', ( #18577, #8039, #3609, #15914 ) ) ;
#12509=CARTESIAN_POINT ( 'NONE',  ( 46.81606138205707168, -37.70325315460876681, 65.37863370302704880 ) ) ;
#12518=CARTESIAN_POINT ( 'NONE',  ( 45.81606138205707168, -38.13418765192403015, 68.51141129791366780 ) ) ;
#12528=CARTESIAN_POINT ( 'NONE',  ( 29.81606138205707879, -39.99575152356569419, 63.13209164280871022 ) ) ;
#12537=ORIENTED_EDGE ( 'NONE', *, *, #20926, .T. ) ;
#12578=FACE_OUTER_BOUND ( 'NONE', #19875, .T. ) ;
#12587=LINE ( 'NONE', #3144, #18984 ) ;
#12593=FACE_OUTER_BOUND ( 'NONE', #6402, .T. ) ;
#12597=DIRECTION ( 'NONE',  ( -1.000000000000000000, -2.999999999999999839E-15, 0.000000000000000000 ) ) ;
#12605=ORIENTED_EDGE ( 'NONE', *, *, #23556, .T. ) ;
#12618=CARTESIAN_POINT ( 'NONE',  ( 40.31606138205701484, -18.06006611532532702, 24.33356453583320445 ) ) ;
#12633=EDGE_CURVE ( 'NONE', #14180, #17786, #23597, .T. ) ;
#12644=CARTESIAN_POINT ( 'NONE',  ( 29.81606138205705037, -30.65246816789535345, 72.44500581826353880 ) ) ;
#12650=LINE ( 'NONE', #20368, #13941 ) ;
#12678=AXIS2_PLACEMENT_3D ( 'NONE', #8011, #15848, #10185 ) ;
#12683=EDGE_CURVE ( 'NONE', #11586, #20703, #13688, .T. ) ;
#12687=VERTEX_POINT ( 'NONE', #14066 ) ;
#12692=ORIENTED_EDGE ( 'NONE', *, *, #7029, .T. ) ;
#12700=AXIS2_PLACEMENT_3D ( 'NONE', #7321, #15428, #1754 ) ;
#12704=DIRECTION ( 'NONE',  ( -1.327674326049719602E-15, 0.4425581086832399147, -0.8967398287344627850 ) ) ;
#12705=DIRECTION ( 'NONE',  ( 2.312964634635742267E-15, -0.8967398287344627850, -0.4425581086832398592 ) ) ;
#12709=ORIENTED_EDGE ( 'NONE', *, *, #523, .F. ) ;
#12719=DIRECTION ( 'NONE',  ( 1.734723475976807094E-15, -0.7516416929448819229, -0.6595716529892350355 ) ) ;
#12722=VECTOR ( 'NONE', #16884, 1000.000000000000114 ) ;
#12724=VERTEX_POINT ( 'NONE', #15866 ) ;
#12727=AXIS2_PLACEMENT_3D ( 'NONE', #863, #10937, #10806 ) ;
#12732=ORIENTED_EDGE ( 'NONE', *, *, #19178, .T. ) ;
#12744=LINE ( 'NONE', #7056, #1211 ) ;
#12758=VERTEX_POINT ( 'NONE', #20623 ) ;
#12761=AXIS2_PLACEMENT_3D ( 'NONE', #16408, #4329, #24256 ) ;
#12766=DIRECTION ( 'NONE',  ( 0.000000000000000000, 0.000000000000000000, 1.000000000000000000 ) ) ;
#12780=AXIS2_PLACEMENT_3D ( 'NONE', #3701, #23535, #7974 ) ;
#12786=LINE ( 'NONE', #8409, #10998 ) ;
#12818=ORIENTED_EDGE ( 'NONE', *, *, #2878, .F. ) ;
#12821=CYLINDRICAL_SURFACE ( 'NONE', #22744, 1.499999999999999778 ) ;
#12828=LINE ( 'NONE', #24637, #23572 ) ;
#12829=VERTEX_POINT ( 'NONE', #18813 ) ;
#12835=ORIENTED_EDGE ( 'NONE', *, *, #6030, .T. ) ;
#12837=DIRECTION ( 'NONE',  ( 1.000000000000000000, 2.999999999999999839E-15, -5.603103565922875308E-33 ) ) ;
#12840=CARTESIAN_POINT ( 'NONE',  ( 46.81606138205697221, -3.984974717493081187, -3.847356352999882656 ) ) ;
#12850=LINE ( 'NONE', #3433, #24657 ) ;
#12873=PLANE ( 'NONE',  #18070 ) ;
#12874=EDGE_CURVE ( 'NONE', #22990, #15655, #12925, .T. ) ;
#12876=CARTESIAN_POINT ( 'NONE',  ( 45.81606138205707168, -38.13418765192403015, 68.51141129791366780 ) ) ;
#12884=AXIS2_PLACEMENT_3D ( 'NONE', #18461, #13871, #4797 ) ;
#12906=EDGE_CURVE ( 'NONE', #5182, #21232, #1785, .T. ) ;
#12918=DIRECTION ( 'NONE',  ( -1.000000000000000000, -2.896293624483393641E-15, 5.118106270778061927E-17 ) ) ;
#12923=DIRECTION ( 'NONE',  ( 1.000000000000000000, 2.999999999999999839E-15, 0.000000000000000000 ) ) ;
#12925=CIRCLE ( 'NONE', #13329, 0.7499999999999996669 ) ;
#12926=CARTESIAN_POINT ( 'NONE',  ( 44.71606138205694947, 3.586515973360805187, -0.5067327973472466329 ) ) ;
#12929=EDGE_CURVE ( 'NONE', #17722, #24841, #20334, .T. ) ;
#12960=EDGE_CURVE ( 'NONE', #16840, #13333, #25225, .T. ) ;
#12962=ADVANCED_FACE ( 'NONE', ( #5285 ), #1287, .T. ) ;
#12965=ORIENTED_EDGE ( 'NONE', *, *, #18708, .T. ) ;
#12991=FACE_OUTER_BOUND ( 'NONE', #8606, .T. ) ;
#13001=DIRECTION ( 'NONE',  ( 1.000000000000000000, 2.999999999999999839E-15, 0.000000000000000000 ) ) ;
#13009=CARTESIAN_POINT ( 'NONE',  ( 36.31606138205702194, -19.40517585842703241, 23.66972737280834238 ) ) ;
#13013=DIRECTION ( 'NONE',  ( -2.417197558325568929E-15, 0.6529557272876933549, 0.7573960774932753104 ) ) ;
#13020=ORIENTED_EDGE ( 'NONE', *, *, #9585, .T. ) ;
#13045=EDGE_CURVE ( 'NONE', #20035, #23539, #12108, .T. ) ;
#13063=AXIS2_PLACEMENT_3D ( 'NONE', #1814, #5690, #21162 ) ;
#13065=CARTESIAN_POINT ( 'NONE',  ( 34.66606138205693810, 6.105630034208187062, 5.871938670042847974 ) ) ;
#13076=ORIENTED_EDGE ( 'NONE', *, *, #10328, .F. ) ;
#13086=VERTEX_POINT ( 'NONE', #25351 ) ;
#13108=VERTEX_POINT ( 'NONE', #21635 ) ;
#13133=EDGE_LOOP ( 'NONE', ( #25269, #8323, #21874, #14956 ) ) ;
#13136=VECTOR ( 'NONE', #1978, 1000.000000000000114 ) ;
#13143=EDGE_CURVE ( 'NONE', #19656, #16125, #7164, .T. ) ;
#13151=AXIS2_PLACEMENT_3D ( 'NONE', #2704, #16365, #22426 ) ;
#13153=DIRECTION ( 'NONE',  ( 2.312964634635742661E-15, -0.4425581086832398037, 0.8967398287344628960 ) ) ;
#13157=VERTEX_POINT ( 'NONE', #23687 ) ;
#13167=EDGE_LOOP ( 'NONE', ( #14246, #6640, #20536, #4103 ) ) ;
#13180=FACE_OUTER_BOUND ( 'NONE', #18096, .T. ) ;
#13201=VERTEX_POINT ( 'NONE', #15018 ) ;
#13204=VECTOR ( 'NONE', #14921, 1000.000000000000000 ) ;
#13209=CARTESIAN_POINT ( 'NONE',  ( 29.81606138205696865, -3.028410647649181442, 0.3252050635115383281 ) ) ;
#13212=FACE_OUTER_BOUND ( 'NONE', #14857, .T. ) ;
#13231=CARTESIAN_POINT ( 'NONE',  ( 44.71606138205697789, -5.918777154956154085, -5.916875169744970187 ) ) ;
#13233=ORIENTED_EDGE ( 'NONE', *, *, #15467, .F. ) ;
#13249=CARTESIAN_POINT ( 'NONE',  ( 41.96606138205694236, 5.651448314156990449, 4.532640732625139002 ) ) ;
#13266=ORIENTED_EDGE ( 'NONE', *, *, #23088, .T. ) ;
#13267=LINE ( 'NONE', #17131, #19976 ) ;
#13281=AXIS2_PLACEMENT_3D ( 'NONE', #12226, #16075, #22009 ) ;
#13282=DIRECTION ( 'NONE',  ( 0.000000000000000000, -0.4425581086832400812, 0.8967398287344626739 ) ) ;
#13301=VECTOR ( 'NONE', #11829, 1000.000000000000000 ) ;
#13312=DIRECTION ( 'NONE',  ( -1.327674326049719602E-15, 0.4425581086832399147, -0.8967398287344627850 ) ) ;
#13329=AXIS2_PLACEMENT_3D ( 'NONE', #8786, #10582, #768 ) ;
#13333=VERTEX_POINT ( 'NONE', #14882 ) ;
#13334=DIRECTION ( 'NONE',  ( -1.327674326049719602E-15, 0.4425581086832399147, -0.8967398287344627850 ) ) ;
#13337=FACE_BOUND ( 'NONE', #17718, .T. ) ;
#13356=ADVANCED_FACE ( 'NONE', ( #8683 ), #5888, .F. ) ;
#13357=DIRECTION ( 'NONE',  ( -1.000000000000000000, -2.952017753711455077E-15, -9.722472704681867976E-17 ) ) ;
#13362=PLANE ( 'NONE',  #4434 ) ;
#13366=ORIENTED_EDGE ( 'NONE', *, *, #3106, .T. ) ;
#13368=DIRECTION ( 'NONE',  ( -1.000000000000000000, -2.999999999999999839E-15, 0.000000000000000000 ) ) ;
#13376=AXIS2_PLACEMENT_3D ( 'NONE', #22766, #1254, #14652 ) ;
#13389=LINE ( 'NONE', #7454, #3313 ) ;
#13398=DIRECTION ( 'NONE',  ( 0.000000000000000000, 0.4425581086832385824, -0.8967398287344634511 ) ) ;
#13401=CARTESIAN_POINT ( 'NONE',  ( 29.81606138205706102, -33.21365173458017495, 70.96885009038120984 ) ) ;
#13404=DIRECTION ( 'NONE',  ( -1.000000000000000000, -2.999999999999999839E-15, 0.000000000000000000 ) ) ;
#13407=ORIENTED_EDGE ( 'NONE', *, *, #7052, .T. ) ;
#13411=ORIENTED_EDGE ( 'NONE', *, *, #24744, .F. ) ;
#13425=LINE ( 'NONE', #15598, #24240 ) ;
#13439=CARTESIAN_POINT ( 'NONE',  ( 42.96606138205694236, 6.105630034208211931, 5.871938670042847974 ) ) ;
#13440=EDGE_CURVE ( 'NONE', #19403, #20407, #23659, .T. ) ;
#13454=CARTESIAN_POINT ( 'NONE',  ( 41.06606138205702194, -19.40517585842701820, 23.66972737280834238 ) ) ;
#13469=CARTESIAN_POINT ( 'NONE',  ( 33.66606138205695231, 3.409598742320806952, 3.426245460917042074 ) ) ;
#13470=CARTESIAN_POINT ( 'NONE',  ( 45.81606138205706458, -34.54722833698617990, 70.28164373264664277 ) ) ;
#13482=ORIENTED_EDGE ( 'NONE', *, *, #25221, .T. ) ;
#13484=CARTESIAN_POINT ( 'NONE',  ( 31.56606138205707168, -38.42645682328038248, 63.90656833300437256 ) ) ;
#13497=AXIS2_PLACEMENT_3D ( 'NONE', #10488, #16136, #22065 ) ;
#13505=EDGE_CURVE ( 'NONE', #22756, #7686, #7957, .T. ) ;
#13516=ORIENTED_EDGE ( 'NONE', *, *, #15663, .F. ) ;
#13533=LINE ( 'NONE', #7616, #23839 ) ;
#13544=FILL_AREA_STYLE_COLOUR ( '', #11852 ) ;
#13574=DIRECTION ( 'NONE',  ( 2.690219486203388234E-15, -0.8967398287344627850, -0.4425581086832399147 ) ) ;
#13578=EDGE_LOOP ( 'NONE', ( #12431, #5778, #16063, #24735 ) ) ;
#13581=DIRECTION ( 'NONE',  ( -2.048868001712899108E-15, 0.6595716529892353686, -0.7516416929448815898 ) ) ;
#13595=EDGE_CURVE ( 'NONE', #21859, #8869, #4242, .T. ) ;
#13601=AXIS2_PLACEMENT_3D ( 'NONE', #14419, #23940, #10060 ) ;
#13603=FACE_OUTER_BOUND ( 'NONE', #23608, .T. ) ;
#13610=DIRECTION ( 'NONE',  ( -2.690219486203388234E-15, 0.8967398287344627850, 0.4425581086832399147 ) ) ;
#13613=ORIENTED_EDGE ( 'NONE', *, *, #623, .F. ) ;
#13617=DIRECTION ( 'NONE',  ( -2.690219486203388234E-15, 0.8967398287344627850, 0.4425581086832399147 ) ) ;
#13627=CARTESIAN_POINT ( 'NONE',  ( 46.81606138205697931, -6.570990706613046406, -2.335727660491067503 ) ) ;
#13629=CARTESIAN_POINT ( 'NONE',  ( 40.56606138205697931, -5.948051402551118194, 9.959574150503843981 ) ) ;
#13632=VERTEX_POINT ( 'NONE', #20032 ) ;
#13635=ORIENTED_EDGE ( 'NONE', *, *, #6858, .F. ) ;
#13636=ORIENTED_EDGE ( 'NONE', *, *, #21945, .F. ) ;
#13639=ORIENTED_EDGE ( 'NONE', *, *, #7068, .T. ) ;
#13646=ORIENTED_EDGE ( 'NONE', *, *, #21829, .F. ) ;
#13655=CARTESIAN_POINT ( 'NONE',  ( 40.31606138205702194, -20.48383445069736197, 23.59578481461660004 ) ) ;
#13657=DIRECTION ( 'NONE',  ( 1.000000000000000000, 0.000000000000000000, 0.000000000000000000 ) ) ;
#13660=ORIENTED_EDGE ( 'NONE', *, *, #18319, .T. ) ;
#13663=ORIENTED_EDGE ( 'NONE', *, *, #623, .T. ) ;
#13669=DIRECTION ( 'NONE',  ( 2.690219486203388234E-15, -0.8967398287344627850, -0.4425581086832399147 ) ) ;
#13679=DIRECTION ( 'NONE',  ( -1.000000000000000000, -3.091505625455828697E-15, -4.515976121274771690E-17 ) ) ;
#13688=LINE ( 'NONE', #386, #16183 ) ;
#13699=EDGE_LOOP ( 'NONE', ( #12168, #20199, #10176, #19750 ) ) ;
#13700=DIRECTION ( 'NONE',  ( -2.515133600231165483E-15, 0.7516416929448815898, 0.6595716529892353686 ) ) ;
#13707=DIRECTION ( 'NONE',  ( 1.000000000000000000, 2.999999999999999839E-15, 0.000000000000000000 ) ) ;
#13708=DIRECTION ( 'NONE',  ( -1.327674326049721180E-15, 0.4425581086832404143, -0.8967398287344625629 ) ) ;
#13718=DIRECTION ( 'NONE',  ( 1.000000000000000000, 2.973811673103095397E-15, 0.000000000000000000 ) ) ;
#13735=ADVANCED_FACE ( 'NONE', ( #18737, #1069 ), #22596, .F. ) ;
#13740=VECTOR ( 'NONE', #20146, 1000.000000000000114 ) ;
#13742=VERTEX_POINT ( 'NONE', #21054 ) ;
#13744=CYLINDRICAL_SURFACE ( 'NONE', #2148, 1.000000000000000888 ) ;
#13752=AXIS2_PLACEMENT_3D ( 'NONE', #23176, #20876, #1651 ) ;
#13765=LINE ( 'NONE', #23153, #15649 ) ;
#13803=CARTESIAN_POINT ( 'NONE',  ( 41.81606138205697221, -2.443590368994772888, -5.798199789213649424 ) ) ;
#13823=CARTESIAN_POINT ( 'NONE',  ( 45.81606138205707879, -39.99575152356564445, 63.13209164280871022 ) ) ;
#13838=ADVANCED_FACE ( 'NONE', ( #6880 ), #12821, .F. ) ;
#13847=CARTESIAN_POINT ( 'NONE',  ( 46.81606138205696510, -2.780187754385526233, -4.367921789353634843 ) ) ;
#13848=ADVANCED_FACE ( 'NONE', ( #5460 ), #9716, .T. ) ;
#13853=ORIENTED_EDGE ( 'NONE', *, *, #3486, .F. ) ;
#13857=PLANE ( 'NONE',  #1522 ) ;
#13871=DIRECTION ( 'NONE',  ( 1.000000000000000000, 2.999999999999999839E-15, 0.000000000000000000 ) ) ;
#13878=DIRECTION ( 'NONE',  ( -3.469446951953614189E-15, 0.8967398287344635621, 0.4425581086832386379 ) ) ;
#13885=DIRECTION ( 'NONE',  ( -1.000000000000000000, -2.999999999999999839E-15, 0.000000000000000000 ) ) ;
#13895=VERTEX_POINT ( 'NONE', #15755 ) ;
#13911=ORIENTED_EDGE ( 'NONE', *, *, #22167, .T. ) ;
#13926=LINE ( 'NONE', #21782, #3603 ) ;
#13929=CARTESIAN_POINT ( 'NONE',  ( 45.81606138205707168, -36.31746077171914067, 73.86860304758450013 ) ) ;
#13935=DIRECTION ( 'NONE',  ( 1.000000000000000000, 3.469446951953611033E-15, 0.000000000000000000 ) ) ;
#13941=VECTOR ( 'NONE', #5168, 1000.000000000000000 ) ;
#13951=DIRECTION ( 'NONE',  ( 1.000000000000000000, 2.999999999999999839E-15, 0.000000000000000000 ) ) ;
#13963=ORIENTED_EDGE ( 'NONE', *, *, #1820, .F. ) ;
#13964=VECTOR ( 'NONE', #4847, 1000.000000000000000 ) ;
#13967=CARTESIAN_POINT ( 'NONE',  ( 31.56606138205697576, -4.349482454670882348, -5.142398479549302515 ) ) ;
#13981=CIRCLE ( 'NONE', #12361, 3.000000000000000888 ) ;
#13994=VERTEX_POINT ( 'NONE', #5840 ) ;
#13996=PLANE ( 'NONE',  #2567 ) ;
#14015=DIRECTION ( 'NONE',  ( -1.000000000000000000, -2.999999999999999839E-15, 0.000000000000000000 ) ) ;
#14019=VERTEX_POINT ( 'NONE', #9839 ) ;
#14031=CARTESIAN_POINT ( 'NONE',  ( 39.31606138205702194, -20.92507021039839543, 32.39841118875936132 ) ) ;
#14037=AXIS2_PLACEMENT_3D ( 'NONE', #15785, #16278, #10369 ) ;
#14051=PLANE ( 'NONE',  #12678 ) ;
#14063=DIRECTION ( 'NONE',  ( 1.225631768639319301E-15, -0.4425581086832399147, 0.8967398287344627850 ) ) ;
#14064=EDGE_CURVE ( 'NONE', #2758, #24942, #2220, .T. ) ;
#14066=CARTESIAN_POINT ( 'NONE',  ( 33.66606138205698073, -6.672912525257909344, -0.4345143786933236552 ) ) ;
#14115=ADVANCED_FACE ( 'NONE', ( #20254 ), #4419, .T. ) ;
#14119=EDGE_LOOP ( 'NONE', ( #17506, #17598, #11686, #2135 ) ) ;
#14126=EDGE_CURVE ( 'NONE', #2216, #20225, #656, .T. ) ;
#14132=EDGE_LOOP ( 'NONE', ( #6037, #7203, #5872, #13020 ) ) ;
#14140=LINE ( 'NONE', #12089, #12294 ) ;
#14141=VECTOR ( 'NONE', #23953, 1000.000000000000000 ) ;
#14153=ORIENTED_EDGE ( 'NONE', *, *, #3089, .T. ) ;
#14158=EDGE_CURVE ( 'NONE', #5343, #24841, #18332, .T. ) ;
#14159=EDGE_CURVE ( 'NONE', #8450, #180, #23730, .T. ) ;
#14161=AXIS2_PLACEMENT_3D ( 'NONE', #8331, #12461, #14499 ) ;
#14167=SURFACE_STYLE_FILL_AREA ( #24783 ) ;
#14180=VERTEX_POINT ( 'NONE', #10601 ) ;
#14188=LINE ( 'NONE', #19981, #14141 ) ;
#14196=VECTOR ( 'NONE', #1052, 1000.000000000000114 ) ;
#14200=EDGE_CURVE ( 'NONE', #18480, #14416, #24832, .T. ) ;
#14214=CARTESIAN_POINT ( 'NONE',  ( 42.96606138205694236, 6.105630034208211931, 5.871938670042847974 ) ) ;
#14239=ORIENTED_EDGE ( 'NONE', *, *, #19349, .F. ) ;
#14242=DIRECTION ( 'NONE',  ( -1.000000000000000000, -2.999999999999999839E-15, 0.000000000000000000 ) ) ;
#14246=ORIENTED_EDGE ( 'NONE', *, *, #19815, .F. ) ;
#14263=CARTESIAN_POINT ( 'NONE',  ( 36.06606138205697931, -5.948051402551132405, 9.959574150503843981 ) ) ;
#14273=CARTESIAN_POINT ( 'NONE',  ( 43.31606138205697221, -3.118133360756952577, 16.65315793475036443 ) ) ;
#14279=AXIS2_PLACEMENT_3D ( 'NONE', #21064, #10646, #18496 ) ;
#14281=EDGE_CURVE ( 'NONE', #19523, #6874, #3463, .T. ) ;
#14284=CARTESIAN_POINT ( 'NONE',  ( 46.81606138205701484, -18.45164032183481595, 27.38658776684409091 ) ) ;
#14285=ADVANCED_FACE ( 'NONE', ( #19180 ), #15051, .T. ) ;
#14299=CARTESIAN_POINT ( 'NONE',  ( 45.81606138205706458, -35.90387122078352178, 69.64117576433150703 ) ) ;
#14316=VECTOR ( 'NONE', #6529, 1000.000000000000000 ) ;
#14327=ORIENTED_EDGE ( 'NONE', *, *, #23246, .T. ) ;
#14334=ORIENTED_EDGE ( 'NONE', *, *, #12929, .T. ) ;
#14336=DIRECTION ( 'NONE',  ( -2.412663730047099099E-15, 0.8967398287344627850, 0.4425581086832399147 ) ) ;
#14345=VERTEX_POINT ( 'NONE', #15437 ) ;
#14359=CARTESIAN_POINT ( 'NONE',  ( 36.06606138205696510, -1.965028424401974227, 1.888915691893686244 ) ) ;
#14380=CARTESIAN_POINT ( 'NONE',  ( 45.81606138205694378, 5.290470704224633280, -0.3848988112044732235 ) ) ;
#14392=ORIENTED_EDGE ( 'NONE', *, *, #9737, .F. ) ;
#14398=EDGE_LOOP ( 'NONE', ( #7282, #940, #12818, #25421, #9173, #18965 ) ) ;
#14410=FACE_OUTER_BOUND ( 'NONE', #11649, .T. ) ;
#14416=VERTEX_POINT ( 'NONE', #3705 ) ;
#14419=CARTESIAN_POINT ( 'NONE',  ( 40.31606138205701484, -20.02093502212014897, 26.61211107664843212 ) ) ;
#14425=LINE ( 'NONE', #4390, #405 ) ;
#14427=CARTESIAN_POINT ( 'NONE',  ( 40.71606138205694947, 3.586515973360791421, -0.5067327973472466329 ) ) ;
#14429=ORIENTED_EDGE ( 'NONE', *, *, #5213, .T. ) ;
#14447=DIRECTION ( 'NONE',  ( 0.000000000000000000, -0.7516416929448823669, -0.6595716529892345914 ) ) ;
#14448=ORIENTED_EDGE ( 'NONE', *, *, #11460, .T. ) ;
#14450=DIRECTION ( 'NONE',  ( -1.225631768639319301E-15, 0.4425581086832399147, -0.8967398287344627850 ) ) ;
#14457=CIRCLE ( 'NONE', #9529, 1.750000000000001998 ) ;
#14461=DIRECTION ( 'NONE',  ( -1.000000000000000000, -2.999999999999999839E-15, 0.000000000000000000 ) ) ;
#14475=VECTOR ( 'NONE', #13951, 1000.000000000000000 ) ;
#14478=LINE ( 'NONE', #18473, #4088 ) ;
#14483=EDGE_CURVE ( 'NONE', #23154, #16840, #1768, .T. ) ;
#14496=CIRCLE ( 'NONE', #20243, 3.000000000000000444 ) ;
#14498=VECTOR ( 'NONE', #23145, 1000.000000000000000 ) ;
#14499=DIRECTION ( 'NONE',  ( -1.225631768639319301E-15, 0.4425581086832399147, -0.8967398287344627850 ) ) ;
#14507=VECTOR ( 'NONE', #2670, 1000.000000000000000 ) ;
#14510=DIRECTION ( 'NONE',  ( -1.123589211228918605E-15, 0.4425581086832399147, -0.8967398287344627850 ) ) ;
#14514=CARTESIAN_POINT ( 'NONE',  ( 36.31606138205701484, -18.91453975041206093, 24.37026150481227305 ) ) ;
#14516=AXIS2_PLACEMENT_3D ( 'NONE', #19275, #25313, #17735 ) ;
#14518=ORIENTED_EDGE ( 'NONE', *, *, #12906, .F. ) ;
#14543=DIRECTION ( 'NONE',  ( 1.000000000000000000, 3.388898908187273079E-15, 1.919289851541777660E-16 ) ) ;
#14552=ORIENTED_EDGE ( 'NONE', *, *, #1302, .F. ) ;
#14569=CARTESIAN_POINT ( 'NONE',  ( 41.96606138205694236, 6.105630034208208379, 5.871938670042847974 ) ) ;
#14593=ORIENTED_EDGE ( 'NONE', *, *, #14621, .F. ) ;
#14601=DIRECTION ( 'NONE',  ( -1.327674326049719602E-15, 0.4425581086832399147, -0.8967398287344627850 ) ) ;
#14606=EDGE_CURVE ( 'NONE', #5217, #4779, #8226, .T. ) ;
#14608=EDGE_LOOP ( 'NONE', ( #23067, #25174 ) ) ;
#14616=ORIENTED_EDGE ( 'NONE', *, *, #14894, .T. ) ;
#14619=CARTESIAN_POINT ( 'NONE',  ( 29.81606138205697221, -3.227578639999851617, -4.500312080287595329 ) ) ;
#14621=EDGE_CURVE ( 'NONE', #2625, #15873, #22254, .T. ) ;
#14622=FACE_OUTER_BOUND ( 'NONE', #11669, .T. ) ;
#14626=CARTESIAN_POINT ( 'NONE',  ( 43.31606138205700063, -14.32738121993773994, 11.12118157620986558 ) ) ;
#14629=ORIENTED_EDGE ( 'NONE', *, *, #25469, .T. ) ;
#14632=EDGE_CURVE ( 'NONE', #20287, #14416, #12026, .T. ) ;
#14635=CARTESIAN_POINT ( 'NONE',  ( 40.71606138205696368, 0.5799492015812739432, -3.145019409304214530 ) ) ;
#14638=CARTESIAN_POINT ( 'NONE',  ( 46.81606138205705747, -33.21365173458013231, 70.96885009038120984 ) ) ;
#14652=DIRECTION ( 'NONE',  ( -3.469446951953616555E-15, 0.8967398287344632291, 0.4425581086832389155 ) ) ;
#14662=ORIENTED_EDGE ( 'NONE', *, *, #7234, .T. ) ;
#14668=CARTESIAN_POINT ( 'NONE',  ( 41.81606138205696510, -1.975699482566714904, -4.057200616784870206 ) ) ;
#14676=CARTESIAN_POINT ( 'NONE',  ( 39.31606138205702194, -21.37925193044962313, 31.05911325134166034 ) ) ;
#14702=CARTESIAN_POINT ( 'NONE',  ( 33.66606138205693810, 6.105630034208183510, 5.871938670042847974 ) ) ;
#14705=EDGE_LOOP ( 'NONE', ( #2512, #20036, #22751, #24218 ) ) ;
#14707=DIRECTION ( 'NONE',  ( 2.792262043613788535E-15, -0.8967398287344627850, -0.4425581086832399147 ) ) ;
#14717=VECTOR ( 'NONE', #23525, 1000.000000000000114 ) ;
#14735=SHAPE_REPRESENTATION ( 'Upper Metal Lever Arm', ( #2000 ), #3041 ) ;
#14749=EDGE_CURVE ( 'NONE', #3879, #22990, #10672, .T. ) ;
#14755=ORIENTED_EDGE ( 'NONE', *, *, #12189, .T. ) ;
#14761=CARTESIAN_POINT ( 'NONE',  ( 36.31606138205697931, -5.528433326023629135, -4.448224773462933435 ) ) ;
#14766=CIRCLE ( 'NONE', #22171, 1.499999999999994005 ) ;
#14771=AXIS2_PLACEMENT_3D ( 'NONE', #3223, #18956, #20885 ) ;
#14780=DIRECTION ( 'NONE',  ( 1.327674326049719602E-15, -0.4425581086832399147, 0.8967398287344627850 ) ) ;
#14788=LINE ( 'NONE', #20722, #20678 ) ;
#14797=EDGE_LOOP ( 'NONE', ( #925, #18975, #24889, #18619 ) ) ;
#14803=DIRECTION ( 'NONE',  ( -1.000000000000000000, -2.751104698760144965E-15, 1.228345504986737969E-16 ) ) ;
#14810=FACE_BOUND ( 'NONE', #20425, .T. ) ;
#14822=EDGE_LOOP ( 'NONE', ( #23501, #896, #6784, #10525 ) ) ;
#14825=CARTESIAN_POINT ( 'NONE',  ( 36.31606138205700063, -14.15704008206721909, 14.73030834591676808 ) ) ;
#14828=ORIENTED_EDGE ( 'NONE', *, *, #2586, .T. ) ;
#14846=PLANE ( 'NONE',  #6488 ) ;
#14857=EDGE_LOOP ( 'NONE', ( #18606, #5156, #7849, #12444 ) ) ;
#14870=ADVANCED_FACE ( 'NONE', ( #22760 ), #7184, .T. ) ;
#14882=CARTESIAN_POINT ( 'NONE',  ( 42.96606138205698500, -7.467730535347522292, -2.778285769174305919 ) ) ;
#14887=ADVANCED_FACE ( 'NONE', ( #3045 ), #5127, .F. ) ;
#14894=EDGE_CURVE ( 'NONE', #12758, #9931, #24676, .T. ) ;
#14917=ORIENTED_EDGE ( 'NONE', *, *, #5824, .T. ) ;
#14921=DIRECTION ( 'NONE',  ( -2.690219486203388234E-15, 0.8967398287344627850, 0.4425581086832399147 ) ) ;
#14928=EDGE_CURVE ( 'NONE', #13108, #17733, #17389, .T. ) ;
#14932=VECTOR ( 'NONE', #12597, 1000.000000000000000 ) ;
#14936=VECTOR ( 'NONE', #15632, 1000.000000000000000 ) ;
#14941=DIRECTION ( 'NONE',  ( -2.792262043613788535E-15, 0.8967398287344627850, 0.4425581086832399147 ) ) ;
#14950=CARTESIAN_POINT ( 'NONE',  ( 46.81606138205696510, -3.028410647649130816, 0.3252050635115383281 ) ) ;
#14956=ORIENTED_EDGE ( 'NONE', *, *, #8386, .F. ) ;
#14991=AXIS2_PLACEMENT_3D ( 'NONE', #25281, #23355, #17707 ) ;
#15000=CARTESIAN_POINT ( 'NONE',  ( 45.81606138205707168, -38.42645682328033985, 63.90656833300437256 ) ) ;
#15002=ORIENTED_EDGE ( 'NONE', *, *, #3996, .T. ) ;
#15003=FACE_OUTER_BOUND ( 'NONE', #10614, .T. ) ;
#15009=ADVANCED_FACE ( 'NONE', ( #8074 ), #13744, .T. ) ;
#15010=VERTEX_POINT ( 'NONE', #21335 ) ;
#15012=DIRECTION ( 'NONE',  ( -1.000000000000000000, -2.999999999999999839E-15, 0.000000000000000000 ) ) ;
#15015=CARTESIAN_POINT ( 'NONE',  ( 34.66606138205693810, 5.651448314156965580, 4.532640732625139002 ) ) ;
#15018=CARTESIAN_POINT ( 'NONE',  ( 30.81606138205697576, -4.349482454670884124, -5.142398479549302515 ) ) ;
#15019=LINE ( 'NONE', #16561, #16854 ) ;
#15025=VECTOR ( 'NONE', #18051, 1000.000000000000000 ) ;
#15036=DIRECTION ( 'NONE',  ( 2.792262043613788535E-15, -0.8967398287344627850, -0.4425581086832399147 ) ) ;
#15037=EDGE_LOOP ( 'NONE', ( #1994, #8663, #11718, #24638 ) ) ;
#15038=CARTESIAN_POINT ( 'NONE',  ( 36.06606138205694378, 4.754708485422509234, 4.090082623941899698 ) ) ;
#15042=LINE ( 'NONE', #20590, #22958 ) ;
#15051=PLANE ( 'NONE',  #481 ) ;
#15059=ORIENTED_EDGE ( 'NONE', *, *, #8500, .T. ) ;
#15061=CARTESIAN_POINT ( 'NONE',  ( 46.81606138205697221, -5.528433326023598049, -4.448224773462933435 ) ) ;
#15067=ADVANCED_FACE ( 'NONE', ( #6136 ), #13996, .F. ) ;
#15076=ORIENTED_EDGE ( 'NONE', *, *, #7059, .F. ) ;
#15090=ORIENTED_EDGE ( 'NONE', *, *, #2786, .T. ) ;
#15103=CIRCLE ( 'NONE', #19624, 1.000000000000000888 ) ;
#15109=EDGE_CURVE ( 'NONE', #9497, #19656, #10379, .T. ) ;
#15119=EDGE_LOOP ( 'NONE', ( #25343, #11143, #4709, #21389 ) ) ;
#15131=PLANE ( 'NONE',  #19207 ) ;
#15140=DIRECTION ( 'NONE',  ( 1.327674326049719602E-15, -0.4425581086832399147, 0.8967398287344627850 ) ) ;
#15143=DIRECTION ( 'NONE',  ( 2.690219486203388234E-15, -0.8967398287344627850, -0.4425581086832399147 ) ) ;
#15146=CIRCLE ( 'NONE', #9389, 1.000000000000000000 ) ;
#15152=CARTESIAN_POINT ( 'NONE',  ( 40.31606138205701484, -20.02093502212014897, 26.61211107664843212 ) ) ;
#15155=EDGE_LOOP ( 'NONE', ( #23193, #9804, #11434, #8378 ) ) ;
#15157=VERTEX_POINT ( 'NONE', #14619 ) ;
#15159=DIRECTION ( 'NONE',  ( -1.000000000000000000, -2.954840238787252245E-15, -9.150562545582958565E-17 ) ) ;
#15188=DIRECTION ( 'NONE',  ( 1.000000000000000000, 2.805550545906362824E-15, -9.596449257708899394E-17 ) ) ;
#15192=CARTESIAN_POINT ( 'NONE',  ( 30.81606138205697576, -3.984974717493129592, -3.847356352999882656 ) ) ;
#15199=LINE ( 'NONE', #25230, #3662 ) ;
#15202=ORIENTED_EDGE ( 'NONE', *, *, #11159, .F. ) ;
#15206=EDGE_CURVE ( 'NONE', #8670, #23160, #4588, .T. ) ;
#15215=EDGE_LOOP ( 'NONE', ( #8702, #23536, #6133, #10003, #17978, #13407, #16509, #12709, #3107, #7025, #21332, #3068, #12009 ) ) ;
#15252=LINE ( 'NONE', #3141, #19114 ) ;
#15254=ORIENTED_EDGE ( 'NONE', *, *, #19815, .T. ) ;
#15260=ORIENTED_EDGE ( 'NONE', *, *, #20449, .T. ) ;
#15268=VERTEX_POINT ( 'NONE', #7150 ) ;
#15269=CYLINDRICAL_SURFACE ( 'NONE', #8593, 0.7500000000000006661 ) ;
#15270=ADVANCED_FACE ( 'NONE', ( #951 ), #5092, .F. ) ;
#15274=ORIENTED_EDGE ( 'NONE', *, *, #4532, .F. ) ;
#15277=EDGE_LOOP ( 'NONE', ( #19882, #20707, #15723, #5836 ) ) ;
#15286=DIRECTION ( 'NONE',  ( 1.327674326049719602E-15, -0.4425581086832399147, 0.8967398287344627850 ) ) ;
#15308=ADVANCED_FACE ( 'NONE', ( #4959 ), #7271, .T. ) ;
#15319=CYLINDRICAL_SURFACE ( 'NONE', #7381, 4.000000000000000000 ) ;
#15336=EDGE_CURVE ( 'NONE', #1959, #5217, #12828, .T. ) ;
#15344=ORIENTED_EDGE ( 'NONE', *, *, #4047, .F. ) ;
#15355=AXIS2_PLACEMENT_3D ( 'NONE', #19592, #1933, #9818 ) ;
#15365=EDGE_CURVE ( 'NONE', #12687, #16840, #11013, .T. ) ;
#15367=ORIENTED_EDGE ( 'NONE', *, *, #23266, .F. ) ;
#15370=DIRECTION ( 'NONE',  ( 2.011972697750610993E-15, -0.6595716529892349245, 0.7516416929448819229 ) ) ;
#15375=ORIENTED_EDGE ( 'NONE', *, *, #14632, .T. ) ;
#15386=ORIENTED_EDGE ( 'NONE', *, *, #24962, .F. ) ;
#15393=CIRCLE ( 'NONE', #4297, 1.749999999999999778 ) ;
#15413=EDGE_CURVE ( 'NONE', #12829, #22022, #628, .T. ) ;
#15428=DIRECTION ( 'NONE',  ( -1.000000000000000000, -2.999999999999999839E-15, 5.603103565922875308E-33 ) ) ;
#15437=CARTESIAN_POINT ( 'NONE',  ( 40.31606138205701484, -19.68901644060771616, 25.93955620509757409 ) ) ;
#15459=ORIENTED_EDGE ( 'NONE', *, *, #23142, .T. ) ;
#15467=EDGE_CURVE ( 'NONE', #4631, #24211, #8772, .T. ) ;
#15468=PRESENTATION_STYLE_ASSIGNMENT (( #3612 ) ) ;
#15476=CARTESIAN_POINT ( 'NONE',  ( 39.31606138205702194, -20.48251210171515879, 31.50167136002490764 ) ) ;
#15492=LINE ( 'NONE', #21558, #2847 ) ;
#15497=CARTESIAN_POINT ( 'NONE',  ( 44.71606138205697079, -4.349482454670842380, -5.142398479549302515 ) ) ;
#15499=CARTESIAN_POINT ( 'NONE',  ( 45.06606138205697221, -4.349482454670840603, -5.142398479549302515 ) ) ;
#15508=VECTOR ( 'NONE', #18820, 1000.000000000000000 ) ;
#15511=EDGE_CURVE ( 'NONE', #24865, #17666, #19240, .T. ) ;
#15516=LINE ( 'NONE', #1355, #20112 ) ;
#15517=DIRECTION ( 'NONE',  ( 2.690219486203388234E-15, -0.8967398287344627850, -0.4425581086832399147 ) ) ;
#15518=CARTESIAN_POINT ( 'NONE',  ( 41.96606138205694947, 5.208890205473748480, 5.429380561359602453 ) ) ;
#15520=ORIENTED_EDGE ( 'NONE', *, *, #8684, .F. ) ;
#15525=FACE_OUTER_BOUND ( 'NONE', #14119, .T. ) ;
#15530=EDGE_CURVE ( 'NONE', #6472, #23154, #19371, .T. ) ;
#15547=CARTESIAN_POINT ( 'NONE',  ( 33.66606138205698073, -5.898435835062239008, -2.003809078978638247 ) ) ;
#15550=DIRECTION ( 'NONE',  ( -1.327674326049719602E-15, 0.4425581086832399147, -0.8967398287344627850 ) ) ;
#15574=DIRECTION ( 'NONE',  ( 3.469446951953570407E-15, -0.8967398287344626739, -0.4425581086832399702 ) ) ;
#15598=CARTESIAN_POINT ( 'NONE',  ( 46.81606138205697221, -5.918777154956146980, -5.916875169744970187 ) ) ;
#15603=FACE_OUTER_BOUND ( 'NONE', #1255, .T. ) ;
#15626=VECTOR ( 'NONE', #3039, 1000.000000000000000 ) ;
#15627=ORIENTED_EDGE ( 'NONE', *, *, #5032, .T. ) ;
#15632=DIRECTION ( 'NONE',  ( 1.000000000000000000, 2.827156040805656045E-15, -8.530177117963464484E-17 ) ) ;
#15636=CIRCLE ( 'NONE', #4534, 4.000000000000000000 ) ;
#15649=VECTOR ( 'NONE', #19173, 1000.000000000000000 ) ;
#15653=VERTEX_POINT ( 'NONE', #23737 ) ;
#15654=DIRECTION ( 'NONE',  ( 1.327674326049719602E-15, -0.4425581086832399147, 0.8967398287344627850 ) ) ;
#15655=VERTEX_POINT ( 'NONE', #4424 ) ;
#15663=EDGE_CURVE ( 'NONE', #22, #12724, #20135, .T. ) ;
#15674=VERTEX_POINT ( 'NONE', #4675 ) ;
#15676=CARTESIAN_POINT ( 'NONE',  ( 30.81606138205696155, -0.2703287878658127696, 1.505452687840413972 ) ) ;
#15695=ORIENTED_EDGE ( 'NONE', *, *, #11804, .F. ) ;
#15697=PLANE ( 'NONE',  #21161 ) ;
#15705=DIRECTION ( 'NONE',  ( 1.000000000000000000, 2.973811673103095397E-15, 0.000000000000000000 ) ) ;
#15706=AXIS2_PLACEMENT_3D ( 'NONE', #24608, #16912, #24741 ) ;
#15723=ORIENTED_EDGE ( 'NONE', *, *, #3442, .F. ) ;
#15738=AXIS2_PLACEMENT_3D ( 'NONE', #1647, #9793, #19433 ) ;
#15740=FACE_OUTER_BOUND ( 'NONE', #17226, .T. ) ;
#15755=CARTESIAN_POINT ( 'NONE',  ( 40.31606138205701484, -19.24645833192448308, 25.04281637636312041 ) ) ;
#15758=ORIENTED_EDGE ( 'NONE', *, *, #23088, .F. ) ;
#15759=FACE_OUTER_BOUND ( 'NONE', #274, .T. ) ;
#15785=CARTESIAN_POINT ( 'NONE',  ( 30.81606138205706458, -34.55876147768187678, 70.30501292735635843 ) ) ;
#15793=ORIENTED_EDGE ( 'NONE', *, *, #24179, .F. ) ;
#15794=DIRECTION ( 'NONE',  ( 1.000000000000000000, 0.000000000000000000, 0.000000000000000000 ) ) ;
#15799=EDGE_CURVE ( 'NONE', #22279, #22756, #1047, .T. ) ;
#15824=EDGE_LOOP ( 'NONE', ( #15520, #34, #13613, #13660, #12311, #5037 ) ) ;
#15837=CARTESIAN_POINT ( 'NONE',  ( 40.31606138205698642, -6.850818256144539653, 29.86554089437370152 ) ) ;
#15848=DIRECTION ( 'NONE',  ( -2.690219486203388234E-15, 0.8967398287344627850, 0.4425581086832399147 ) ) ;
#15865=EDGE_CURVE ( 'NONE', #2738, #5929, #3369, .T. ) ;
#15866=CARTESIAN_POINT ( 'NONE',  ( 30.81606138205706813, -35.90867894478445521, 74.07034463014319670 ) ) ;
#15873=VERTEX_POINT ( 'NONE', #2976 ) ;
#15877=CARTESIAN_POINT ( 'NONE',  ( 30.81606138205694378, 5.290470704224592424, -0.3848988112044732235 ) ) ;
#15890=FACE_OUTER_BOUND ( 'NONE', #23606, .T. ) ;
#15892=EDGE_CURVE ( 'NONE', #12198, #14019, #21138, .T. ) ;
#15898=DIRECTION ( 'NONE',  ( -1.000000000000000000, -3.091505625455828697E-15, -4.515976121274772923E-17 ) ) ;
#15903=EDGE_CURVE ( 'NONE', #7024, #19403, #5052, .T. ) ;
#15905=ORIENTED_EDGE ( 'NONE', *, *, #1072, .F. ) ;
#15914=ORIENTED_EDGE ( 'NONE', *, *, #6723, .F. ) ;
#15918=CIRCLE ( 'NONE', #22503, 1.499999999999999778 ) ;
#15921=DIRECTION ( 'NONE',  ( 3.965082230804126670E-15, -0.8967398287344626739, -0.4425581086832401922 ) ) ;
#15934=CIRCLE ( 'NONE', #8124, 4.000000000000000000 ) ;
#15945=LINE ( 'NONE', #4113, #7116 ) ;
#15989=CARTESIAN_POINT ( 'NONE',  ( 33.66606138205693810, 6.105630034208183510, 5.871938670042847974 ) ) ;
#16002=EDGE_LOOP ( 'NONE', ( #13963, #18665, #4838, #20241 ) ) ;
#16005=CARTESIAN_POINT ( 'NONE',  ( 30.81606138205709300, -43.53621639303160862, 70.30601027268440362 ) ) ;
#16018=CARTESIAN_POINT ( 'NONE',  ( 45.81606138205707168, -36.80651332587431313, 65.82119181171029254 ) ) ;
#16036=VECTOR ( 'NONE', #15898, 1000.000000000000000 ) ;
#16049=DIRECTION ( 'NONE',  ( 1.000000000000000000, 2.999999999999999839E-15, -5.603103565922875308E-33 ) ) ;
#16055=ADVANCED_FACE ( 'NONE', ( #21154 ), #7629, .T. ) ;
#16057=FACE_OUTER_BOUND ( 'NONE', #22057, .T. ) ;
#16058=VECTOR ( 'NONE', #18270, 1000.000000000000000 ) ;
#16063=ORIENTED_EDGE ( 'NONE', *, *, #20498, .F. ) ;
#16066=ORIENTED_EDGE ( 'NONE', *, *, #15903, .F. ) ;
#16070=ORIENTED_EDGE ( 'NONE', *, *, #15365, .T. ) ;
#16075=DIRECTION ( 'NONE',  ( 1.327674326049719602E-15, -0.4425581086832399147, 0.8967398287344627850 ) ) ;
#16078=PLANE ( 'NONE',  #1157 ) ;
#16079=EDGE_CURVE ( 'NONE', #7819, #16874, #21654, .T. ) ;
#16084=DIRECTION ( 'NONE',  ( 1.327674326049719602E-15, -0.4425581086832399147, 0.8967398287344627850 ) ) ;
#16085=AXIS2_PLACEMENT_3D ( 'NONE', #17490, #17106, #25315 ) ;
#16090=EDGE_CURVE ( 'NONE', #5182, #20407, #9319, .T. ) ;
#16125=VERTEX_POINT ( 'NONE', #2566 ) ;
#16131=DIRECTION ( 'NONE',  ( -2.690219486203388234E-15, 0.8967398287344627850, 0.4425581086832399147 ) ) ;
#16136=DIRECTION ( 'NONE',  ( 1.000000000000000000, 3.001186103030333510E-15, 2.281710121244060993E-16 ) ) ;
#16140=DIRECTION ( 'NONE',  ( -1.327674326049719602E-15, 0.4425581086832399147, -0.8967398287344627850 ) ) ;
#16148=CARTESIAN_POINT ( 'NONE',  ( 40.71606138205694947, 3.586515973360791421, -0.5067327973472466329 ) ) ;
#16153=EDGE_LOOP ( 'NONE', ( #25069, #15002, #18860, #15386 ) ) ;
#16155=DIRECTION ( 'NONE',  ( -1.000000000000000000, -2.999999999999999839E-15, 0.000000000000000000 ) ) ;
#16161=ORIENTED_EDGE ( 'NONE', *, *, #15865, .T. ) ;
#16170=EDGE_CURVE ( 'NONE', #24865, #17786, #14188, .T. ) ;
#16180=CARTESIAN_POINT ( 'NONE',  ( 45.81606138205705747, -32.32696853385078128, 75.83798663122490780 ) ) ;
#16183=VECTOR ( 'NONE', #8272, 1000.000000000000000 ) ;
#16186=CARTESIAN_POINT ( 'NONE',  ( 46.81606138205707168, -35.90867894478441258, 74.07034463014319670 ) ) ;
#16188=ADVANCED_FACE ( 'NONE', ( #21907 ), #248, .F. ) ;
#16194=ORIENTED_EDGE ( 'NONE', *, *, #24899, .T. ) ;
#16201=FACE_BOUND ( 'NONE', #3202, .T. ) ;
#16202=CIRCLE ( 'NONE', #5113, 1.750000000000001998 ) ;
#16208=FILL_AREA_STYLE_COLOUR ( '', #17873 ) ;
#16216=ORIENTED_EDGE ( 'NONE', *, *, #10186, .T. ) ;
#16245=FACE_OUTER_BOUND ( 'NONE', #13699, .T. ) ;
#16263=CARTESIAN_POINT ( 'NONE',  ( 30.81606138205705747, -33.21365173458017495, 70.96885009038120984 ) ) ;
#16278=DIRECTION ( 'NONE',  ( 1.000000000000000000, 2.999999999999999839E-15, 0.000000000000000000 ) ) ;
#16280=ORIENTED_EDGE ( 'NONE', *, *, #22996, .F. ) ;
#16282=DIRECTION ( 'NONE',  ( -4.625929269271484533E-15, 0.8967398287344634511, 0.4425581086832385824 ) ) ;
#16300=DIRECTION ( 'NONE',  ( -2.690219486203388234E-15, 0.8967398287344627850, 0.4425581086832399147 ) ) ;
#16302=CARTESIAN_POINT ( 'NONE',  ( 36.31606138205702194, -19.24645833192449373, 25.04281637636312041 ) ) ;
#16303=CARTESIAN_POINT ( 'NONE',  ( 40.31606138205702194, -21.82181003913286332, 31.95585308007613179 ) ) ;
#16310=CARTESIAN_POINT ( 'NONE',  ( 36.06606138205696510, -1.522470315718732037, 0.9921758631592225708 ) ) ;
#16315=ORIENTED_EDGE ( 'NONE', *, *, #8820, .F. ) ;
#16334=FACE_OUTER_BOUND ( 'NONE', #16153, .T. ) ;
#16350=EDGE_CURVE ( 'NONE', #24211, #20287, #8771, .T. ) ;
#16357=CARTESIAN_POINT ( 'NONE',  ( 45.81606138205697221, -4.349482454670838827, -5.142398479549302515 ) ) ;
#16365=DIRECTION ( 'NONE',  ( -1.327674326049719602E-15, 0.4425581086832399147, -0.8967398287344627850 ) ) ;
#16373=DIRECTION ( 'NONE',  ( -2.690219486203388234E-15, 0.8967398287344627850, 0.4425581086832399147 ) ) ;
#16374=DIRECTION ( 'NONE',  ( 1.000000000000000000, 3.091505625455828697E-15, 4.515976121274736561E-17 ) ) ;
#16376=ORIENTED_EDGE ( 'NONE', *, *, #10317, .T. ) ;
#16404=EDGE_CURVE ( 'NONE', #2906, #16878, #3031, .T. ) ;
#16408=CARTESIAN_POINT ( 'NONE',  ( 30.81606138205697576, -4.349482454670884124, -5.142398479549302515 ) ) ;
#16413=ORIENTED_EDGE ( 'NONE', *, *, #11318, .F. ) ;
#16426=VECTOR ( 'NONE', #17685, 1000.000000000000000 ) ;
#16427=DIRECTION ( 'NONE',  ( -1.000000000000000000, -2.999999999999999839E-15, 0.000000000000000000 ) ) ;
#16451=CARTESIAN_POINT ( 'NONE',  ( 38.31606138205694378, 3.409598742320820719, 3.426245460917042074 ) ) ;
#16472=DIRECTION ( 'NONE',  ( 1.000000000000000000, 2.999999999999999839E-15, 0.000000000000000000 ) ) ;
#16500=VERTEX_POINT ( 'NONE', #17132 ) ;
#16509=ORIENTED_EDGE ( 'NONE', *, *, #14126, .F. ) ;
#16523=VECTOR ( 'NONE', #10545, 1000.000000000000000 ) ;
#16535=DIRECTION ( 'NONE',  ( -2.412663730047099099E-15, 0.8967398287344627850, 0.4425581086832399147 ) ) ;
#16540=ORIENTED_EDGE ( 'NONE', *, *, #4207, .F. ) ;
#16551=ORIENTED_EDGE ( 'NONE', *, *, #19399, .F. ) ;
#16561=CARTESIAN_POINT ( 'NONE',  ( 36.31606138205702905, -21.82181003913287398, 31.95585308007613179 ) ) ;
#16564=DIRECTION ( 'NONE',  ( -2.048868001712896742E-15, 0.6595716529892345914, -0.7516416929448823669 ) ) ;
#16576=DIRECTION ( 'NONE',  ( 2.312964634635742267E-15, -0.8967398287344627850, -0.4425581086832398592 ) ) ;
#16583=CARTESIAN_POINT ( 'NONE',  ( 34.66606138205694521, 5.208890205473723611, 5.429380561359602453 ) ) ;
#16598=ORIENTED_EDGE ( 'NONE', *, *, #21995, .T. ) ;
#16603=CARTESIAN_POINT ( 'NONE',  ( 31.91606138205697718, -5.022037326221728826, -5.474317061061731771 ) ) ;
#16621=VECTOR ( 'NONE', #24773, 1000.000000000000000 ) ;
#16637=DIRECTION ( 'NONE',  ( -2.574571254471601357E-15, 0.8967398287344627850, 0.4425581086832399147 ) ) ;
#16638=EDGE_CURVE ( 'NONE', #12758, #21730, #17254, .T. ) ;
#16639=AXIS2_PLACEMENT_3D ( 'NONE', #18088, #14461, #16131 ) ;
#16642=EDGE_CURVE ( 'NONE', #6874, #22610, #10040, .T. ) ;
#16648=AXIS2_PLACEMENT_3D ( 'NONE', #21034, #21160, #18584 ) ;
#16675=ADVANCED_FACE ( 'NONE', ( #22479 ), #15697, .T. ) ;
#16681=ORIENTED_EDGE ( 'NONE', *, *, #24048, .T. ) ;
#16689=DIRECTION ( 'NONE',  ( -1.327674326049719602E-15, 0.4425581086832399147, -0.8967398287344627850 ) ) ;
#16693=SURFACE_SIDE_STYLE ('',( #14167 ) ) ;
#16701=ORIENTED_EDGE ( 'NONE', *, *, #1667, .T. ) ;
#16704=DIRECTION ( 'NONE',  ( -1.000000000000000000, -3.091505625455829092E-15, -4.515976121274730398E-17 ) ) ;
#16714=DIRECTION ( 'NONE',  ( 1.000000000000000000, 2.999999999999999839E-15, 0.000000000000000000 ) ) ;
#16717=EDGE_CURVE ( 'NONE', #24103, #15157, #3865, .T. ) ;
#16722=ADVANCED_FACE ( 'NONE', ( #23545 ), #22356, .F. ) ;
#16735=DIRECTION ( 'NONE',  ( 2.690219486203388234E-15, -0.8967398287344627850, -0.4425581086832399147 ) ) ;
#16752=LINE ( 'NONE', #22556, #23812 ) ;
#16759=EDGE_CURVE ( 'NONE', #22610, #1644, #16202, .T. ) ;
#16772=PLANE ( 'NONE',  #15706 ) ;
#16774=CARTESIAN_POINT ( 'NONE',  ( 46.81606138205707168, -35.90387122078352178, 69.64117576433150703 ) ) ;
#16779=AXIS2_PLACEMENT_3D ( 'NONE', #24611, #2984, #923 ) ;
#16781=LINE ( 'NONE', #12432, #12503 ) ;
#16783=DIRECTION ( 'NONE',  ( 0.000000000000000000, -0.4425581086832348077, 0.8967398287344653385 ) ) ;
#16804=DIRECTION ( 'NONE',  ( 2.690219486203388234E-15, -0.8967398287344627850, -0.4425581086832399147 ) ) ;
#16813=VECTOR ( 'NONE', #13708, 1000.000000000000000 ) ;
#16833=ORIENTED_EDGE ( 'NONE', *, *, #13505, .T. ) ;
#16840=VERTEX_POINT ( 'NONE', #17200 ) ;
#16854=VECTOR ( 'NONE', #20320, 1000.000000000000000 ) ;
#16858=PLANE ( 'NONE',  #12727 ) ;
#16871=EDGE_CURVE ( 'NONE', #5334, #20374, #19130, .T. ) ;
#16872=CARTESIAN_POINT ( 'NONE',  ( 41.06606138205702194, -20.30191568716147898, 23.22716926412510219 ) ) ;
#16874=VERTEX_POINT ( 'NONE', #24896 ) ;
#16878=VERTEX_POINT ( 'NONE', #21190 ) ;
#16884=DIRECTION ( 'NONE',  ( -2.011972697750612571E-15, 0.6595716529892353686, -0.7516416929448815898 ) ) ;
#16908=CARTESIAN_POINT ( 'NONE',  ( 45.81606138205707168, -37.70325315460877391, 65.37863370302704880 ) ) ;
#16912=DIRECTION ( 'NONE',  ( 1.169972191870009723E-15, -0.4425581086832399147, 0.8967398287344627850 ) ) ;
#16929=VERTEX_POINT ( 'NONE', #13454 ) ;
#16936=DIRECTION ( 'NONE',  ( 2.792262043613788930E-15, -0.8967398287344627850, -0.4425581086832399147 ) ) ;
#16955=LINE ( 'NONE', #11033, #13964 ) ;
#16959=ORIENTED_EDGE ( 'NONE', *, *, #10328, .T. ) ;
#16979=CARTESIAN_POINT ( 'NONE',  ( 29.81606138205706813, -35.90387122078357152, 69.64117576433150703 ) ) ;
#17022=EDGE_CURVE ( 'NONE', #8670, #23228, #22805, .T. ) ;
#17044=LINE ( 'NONE', #7248, #14196 ) ;
#17049=FACE_OUTER_BOUND ( 'NONE', #7752, .T. ) ;
#17058=CARTESIAN_POINT ( 'NONE',  ( 46.81606138205707879, -38.42645682328033274, 63.90656833300437256 ) ) ;
#17071=ORIENTED_EDGE ( 'NONE', *, *, #24179, .T. ) ;
#17089=LINE ( 'NONE', #24907, #13136 ) ;
#17090=CARTESIAN_POINT ( 'NONE',  ( 34.81606138205696510, -0.8482369431493941292, -3.067843137301039302 ) ) ;
#17094=DIRECTION ( 'NONE',  ( 1.000000000000000000, 2.751104698760144965E-15, -1.228345504986737969E-16 ) ) ;
#17104=DIRECTION ( 'NONE',  ( 1.000000000000000000, 2.751104698760144965E-15, -1.228345504986737969E-16 ) ) ;
#17106=DIRECTION ( 'NONE',  ( 1.000000000000000000, 2.999999999999999839E-15, 0.000000000000000000 ) ) ;
#17110=VERTEX_POINT ( 'NONE', #16263 ) ;
#17131=CARTESIAN_POINT ( 'NONE',  ( 46.81606138205697221, -5.022037326221683529, -5.474317061061731771 ) ) ;
#17132=CARTESIAN_POINT ( 'NONE',  ( 36.31606138205702194, -19.68901644060773037, 25.93955620509758475 ) ) ;
#17137=LINE ( 'NONE', #5281, #19496 ) ;
#17149=ORIENTED_EDGE ( 'NONE', *, *, #7059, .T. ) ;
#17159=VECTOR ( 'NONE', #14450, 1000.000000000000000 ) ;
#17178=CIRCLE ( 'NONE', #18411, 1.000000000000000888 ) ;
#17200=CARTESIAN_POINT ( 'NONE',  ( 42.96606138205698500, -6.672912525257881811, -0.4345143786933236552 ) ) ;
#17201=DIRECTION ( 'NONE',  ( 2.312964634635742267E-15, -0.8967398287344634511, -0.4425581086832385824 ) ) ;
#17221=EDGE_LOOP ( 'NONE', ( #11542, #15090, #2746, #13366 ) ) ;
#17226=EDGE_LOOP ( 'NONE', ( #5408, #1888, #21772, #23043 ) ) ;
#17233=CARTESIAN_POINT ( 'NONE',  ( 35.91606138205695231, 2.926944320371551278, 0.2449088955976189141 ) ) ;
#17239=VECTOR ( 'NONE', #4253, 1000.000000000000000 ) ;
#17241=ORIENTED_EDGE ( 'NONE', *, *, #24414, .T. ) ;
#17249=CARTESIAN_POINT ( 'NONE',  ( 46.81606138205695800, -0.2703287878657641974, 1.505452687840413972 ) ) ;
#17254=LINE ( 'NONE', #22913, #12111 ) ;
#17257=CIRCLE ( 'NONE', #24236, 1.499999999999999778 ) ;
#17259=CARTESIAN_POINT ( 'NONE',  ( 30.81606138205706102, -34.13844651005150155, 70.48338531520533934 ) ) ;
#17274=CIRCLE ( 'NONE', #22621, 1.499999999999999778 ) ;
#17278=VECTOR ( 'NONE', #18182, 1000.000000000000000 ) ;
#17279=EDGE_LOOP ( 'NONE', ( #11465, #25334, #19090, #12446 ) ) ;
#17285=ORIENTED_EDGE ( 'NONE', *, *, #10191, .F. ) ;
#17289=ADVANCED_FACE ( 'NONE', ( #9068 ), #16772, .F. ) ;
#17295=DIRECTION ( 'NONE',  ( -1.047880217021202589E-15, 0.4425581086832399147, -0.8967398287344627850 ) ) ;
#17299=PLANE ( 'NONE',  #4828 ) ;
#17302=SHAPE_DEFINITION_REPRESENTATION ( #21867, #14735 ) ;
#17327=EDGE_LOOP ( 'NONE', ( #15260, #3819, #2868, #21964 ) ) ;
#17332=DIRECTION ( 'NONE',  ( 1.327674326049719602E-15, -0.4425581086832399147, 0.8967398287344627850 ) ) ;
#17352=DIRECTION ( 'NONE',  ( -1.000000000000000000, -3.091505625455828697E-15, -4.515976121274771690E-17 ) ) ;
#17360=CARTESIAN_POINT ( 'NONE',  ( 30.81606138205697576, -4.349482454670884124, -5.142398479549302515 ) ) ;
#17364=AXIS2_PLACEMENT_3D ( 'NONE', #2788, #8874, #9131 ) ;
#17366=EDGE_CURVE ( 'NONE', #13895, #22610, #21158, .T. ) ;
#17368=EDGE_CURVE ( 'NONE', #7931, #11230, #19724, .T. ) ;
#17369=VERTEX_POINT ( 'NONE', #13803 ) ;
#17389=CIRCLE ( 'NONE', #14516, 4.000000000000000000 ) ;
#17406=ORIENTED_EDGE ( 'NONE', *, *, #7043, .T. ) ;
#17411=VECTOR ( 'NONE', #4346, 1000.000000000000000 ) ;
#17415=EDGE_CURVE ( 'NONE', #15653, #8578, #6573, .T. ) ;
#17418=CARTESIAN_POINT ( 'NONE',  ( 45.06606138205697931, -5.918777154956152309, -5.916875169744970187 ) ) ;
#17424=DIRECTION ( 'NONE',  ( -1.000000000000000000, -2.999999999999999839E-15, 0.000000000000000000 ) ) ;
#17465=VECTOR ( 'NONE', #8957, 1000.000000000000000 ) ;
#17471=DIRECTION ( 'NONE',  ( 1.327674326049719602E-15, -0.4425581086832399147, 0.8967398287344627850 ) ) ;
#17484=ORIENTED_EDGE ( 'NONE', *, *, #24182, .T. ) ;
#17488=ORIENTED_EDGE ( 'NONE', *, *, #25452, .T. ) ;
#17490=CARTESIAN_POINT ( 'NONE',  ( 42.96606138205697789, -5.898435835062210586, -2.003809078978638247 ) ) ;
#17506=ORIENTED_EDGE ( 'NONE', *, *, #5240, .F. ) ;
#17521=DIRECTION ( 'NONE',  ( 2.602085213965210642E-15, -0.8967398287344635621, -0.4425581086832386379 ) ) ;
#17532=ADVANCED_FACE ( 'NONE', ( #12261, #2444 ), #10320, .F. ) ;
#17533=LINE ( 'NONE', #5932, #387 ) ;
#17535=EDGE_LOOP ( 'NONE', ( #6896, #11313, #4218, #10942 ) ) ;
#17544=ORIENTED_EDGE ( 'NONE', *, *, #2860, .T. ) ;
#17548=DIRECTION ( 'NONE',  ( -1.000000000000000000, -3.091505625455828697E-15, -4.515976121274772923E-17 ) ) ;
#17570=ORIENTED_EDGE ( 'NONE', *, *, #24517, .T. ) ;
#17571=CARTESIAN_POINT ( 'NONE',  ( 37.31606138205698642, -10.17000407126884376, 36.59108960988216808 ) ) ;
#17583=AXIS2_PLACEMENT_3D ( 'NONE', #23749, #23993, #16140 ) ;
#17586=LINE ( 'NONE', #23362, #23722 ) ;
#17595=ORIENTED_EDGE ( 'NONE', *, *, #1368, .T. ) ;
#17598=ORIENTED_EDGE ( 'NONE', *, *, #523, .T. ) ;
#17605=ORIENTED_EDGE ( 'NONE', *, *, #11381, .T. ) ;
#17611=EDGE_CURVE ( 'NONE', #19039, #10246, #1716, .T. ) ;
#17613=CARTESIAN_POINT ( 'NONE',  ( 29.81606138205696865, -3.028410647649181442, 0.3252050635115383281 ) ) ;
#17619=CARTESIAN_POINT ( 'NONE',  ( 45.06606138205707879, -38.42645682328033985, 63.90656833300437256 ) ) ;
#17625=CIRCLE ( 'NONE', #21309, 1.000000000000011990 ) ;
#17631=EDGE_LOOP ( 'NONE', ( #7739, #6476, #15627, #445 ) ) ;
#17642=DIRECTION ( 'NONE',  ( -1.000000000000000000, -2.999999999999999839E-15, 0.000000000000000000 ) ) ;
#17659=VERTEX_POINT ( 'NONE', #12644 ) ;
#17666=VERTEX_POINT ( 'NONE', #4229 ) ;
#17680=FACE_OUTER_BOUND ( 'NONE', #18492, .T. ) ;
#17685=DIRECTION ( 'NONE',  ( 2.442401846778130416E-15, -0.8967398287344627850, -0.4425581086832399147 ) ) ;
#17694=ORIENTED_EDGE ( 'NONE', *, *, #10049, .T. ) ;
#17702=CARTESIAN_POINT ( 'NONE',  ( 33.66606138205698073, -6.230354416574667376, -1.331254207427787328 ) ) ;
#17703=ORIENTED_EDGE ( 'NONE', *, *, #19083, .F. ) ;
#17704=CARTESIAN_POINT ( 'NONE',  ( 46.81606138205697931, -6.570990706613046406, -2.335727660491067503 ) ) ;
#17707=DIRECTION ( 'NONE',  ( 0.000000000000000000, -0.7516416929448823669, -0.6595716529892345914 ) ) ;
#17718=EDGE_LOOP ( 'NONE', ( #9762, #24187 ) ) ;
#17722=VERTEX_POINT ( 'NONE', #2775 ) ;
#17733=VERTEX_POINT ( 'NONE', #4485 ) ;
#17735=DIRECTION ( 'NONE',  ( 1.734723475976807094E-15, -0.7516416929448819229, -0.6595716529892350355 ) ) ;
#17757=LINE ( 'NONE', #21619, #1638 ) ;
#17780=CARTESIAN_POINT ( 'NONE',  ( 36.31606138205702194, -21.37925193044963379, 31.05911325134166034 ) ) ;
#17786=VERTEX_POINT ( 'NONE', #16310 ) ;
#17799=FACE_OUTER_BOUND ( 'NONE', #22000, .T. ) ;
#17803=VECTOR ( 'NONE', #6540, 1000.000000000000000 ) ;
#17805=DIRECTION ( 'NONE',  ( 1.000000000000000000, 3.217519435284891566E-15, 1.466282614970859239E-16 ) ) ;
#17815=AXIS2_PLACEMENT_3D ( 'NONE', #8341, #4349, #16300 ) ;
#17821=CARTESIAN_POINT ( 'NONE',  ( 31.91606138205697363, -4.349482454670880571, -5.142398479549302515 ) ) ;
#17873=COLOUR_RGB ( '', 0.09019608, 0.27058824, 0.51372549) ;
#17879=EDGE_LOOP ( 'NONE', ( #3355, #18330, #15059, #18662 ) ) ;
#17882=VECTOR ( 'NONE', #13013, 1000.000000000000000 ) ;
#17885=FACE_OUTER_BOUND ( 'NONE', #1639, .T. ) ;
#17887=CARTESIAN_POINT ( 'NONE',  ( 39.31606138205702194, -21.82181003913286332, 31.95585308007613179 ) ) ;
#17890=ORIENTED_EDGE ( 'NONE', *, *, #11386, .T. ) ;
#17896=VECTOR ( 'NONE', #22853, 1000.000000000000000 ) ;
#17905=CARTESIAN_POINT ( 'NONE',  ( 46.81606138205706458, -34.55876147768182705, 70.30501292735635843 ) ) ;
#17929=EDGE_LOOP ( 'NONE', ( #2959, #23284 ) ) ;
#17930=LINE ( 'NONE', #8391, #15025 ) ;
#17931=DIRECTION ( 'NONE',  ( 1.000000000000000000, 2.999999999999999839E-15, 0.000000000000000000 ) ) ;
#17956=DIRECTION ( 'NONE',  ( 0.000000000000000000, -0.4425581086832361399, 0.8967398287344645613 ) ) ;
#17959=ADVANCED_FACE ( 'NONE', ( #18638 ), #18767, .F. ) ;
#17961=PLANE ( 'NONE',  #16639 ) ;
#17975=CARTESIAN_POINT ( 'NONE',  ( 42.96606138205697789, -6.230354416574639842, -1.331254207427787328 ) ) ;
#17978=ORIENTED_EDGE ( 'NONE', *, *, #23684, .T. ) ;
#17985=UNCERTAINTY_MEASURE_WITH_UNIT (LENGTH_MEASURE( 1.000000000000000082E-05 ), #4006, 'distance_accuracy_value', 'NONE');
#17989=ORIENTED_EDGE ( 'NONE', *, *, #10191, .T. ) ;
#17993=ORIENTED_EDGE ( 'NONE', *, *, #8713, .T. ) ;
#18030=DIRECTION ( 'NONE',  ( -1.327674326049719602E-15, 0.4425581086832399147, -0.8967398287344627850 ) ) ;
#18035=CARTESIAN_POINT ( 'NONE',  ( 45.06606138205707879, -39.99575152356565155, 63.13209164280871022 ) ) ;
#18041=CARTESIAN_POINT ( 'NONE',  ( 46.81606138205707168, -36.80651332587431313, 65.82119181171029254 ) ) ;
#18051=DIRECTION ( 'NONE',  ( 2.690219486203388234E-15, -0.8967398287344627850, -0.4425581086832399147 ) ) ;
#18052=DIRECTION ( 'NONE',  ( 1.000000000000000000, 3.469446951953611033E-15, 0.000000000000000000 ) ) ;
#18062=CARTESIAN_POINT ( 'NONE',  ( 36.31606138205702194, -20.02093502212016318, 26.61211107664843212 ) ) ;
#18070=AXIS2_PLACEMENT_3D ( 'NONE', #9010, #13001, #11063 ) ;
#18080=EDGE_CURVE ( 'NONE', #12198, #20897, #9871, .T. ) ;
#18081=DIRECTION ( 'NONE',  ( 1.327674326049719602E-15, -0.4425581086832399147, 0.8967398287344627850 ) ) ;
#18088=CARTESIAN_POINT ( 'NONE',  ( 42.96606138205697789, -5.898435835062210586, -2.003809078978638247 ) ) ;
#18096=EDGE_LOOP ( 'NONE', ( #6797, #16315, #10670, #6306 ) ) ;
#18101=CARTESIAN_POINT ( 'NONE',  ( 31.56606138205697576, -4.349482454670882348, -5.142398479549302515 ) ) ;
#18114=LINE ( 'NONE', #8572, #7403 ) ;
#18126=CYLINDRICAL_SURFACE ( 'NONE', #18407, 1.750000000000001776 ) ;
#18131=VECTOR ( 'NONE', #6980, 1000.000000000000000 ) ;
#18133=CARTESIAN_POINT ( 'NONE',  ( 41.96606138205694236, 6.548188142891450347, 4.975198841308384523 ) ) ;
#18138=ADVANCED_FACE ( 'NONE', ( #21208 ), #13857, .F. ) ;
#18139=ADVANCED_FACE ( 'NONE', ( #15525 ), #13362, .T. ) ;
#18140=DIRECTION ( 'NONE',  ( 2.792262043613788535E-15, -0.8967398287344627850, -0.4425581086832399147 ) ) ;
#18144=VERTEX_POINT ( 'NONE', #19650 ) ;
#18170=VERTEX_POINT ( 'NONE', #2796 ) ;
#18177=LINE ( 'NONE', #22151, #16813 ) ;
#18182=DIRECTION ( 'NONE',  ( 2.412663730047099099E-15, -0.8967398287344627850, -0.4425581086832399147 ) ) ;
#18183=CARTESIAN_POINT ( 'NONE',  ( 46.81606138205695089, 5.290470704224636833, -0.3848988112044732235 ) ) ;
#18213=DIRECTION ( 'NONE',  ( 0.000000000000000000, -0.4425581086832404143, 0.8967398287344625629 ) ) ;
#18227=VECTOR ( 'NONE', #4492, 1000.000000000000000 ) ;
#18231=ORIENTED_EDGE ( 'NONE', *, *, #15206, .T. ) ;
#18237=DIRECTION ( 'NONE',  ( -1.000000000000000000, -2.999999999999999839E-15, 0.000000000000000000 ) ) ;
#18253=ORIENTED_EDGE ( 'NONE', *, *, #21926, .T. ) ;
#18254=ORIENTED_EDGE ( 'NONE', *, *, #20187, .T. ) ;
#18270=DIRECTION ( 'NONE',  ( -2.412663730047099099E-15, 0.8967398287344627850, 0.4425581086832399147 ) ) ;
#18294=ORIENTED_EDGE ( 'NONE', *, *, #24517, .F. ) ;
#18304=ADVANCED_FACE ( 'NONE', ( #4871, #22646, #14410 ), #8879, .F. ) ;
#18307=VERTEX_POINT ( 'NONE', #4622 ) ;
#18318=DIRECTION ( 'NONE',  ( 0.000000000000000000, -0.4425581086832348077, 0.8967398287344653385 ) ) ;
#18319=EDGE_CURVE ( 'NONE', #5929, #3431, #17178, .T. ) ;
#18323=DIRECTION ( 'NONE',  ( -2.602085213965212219E-15, 0.8967398287344632291, 0.4425581086832389155 ) ) ;
#18328=ORIENTED_EDGE ( 'NONE', *, *, #17022, .F. ) ;
#18330=ORIENTED_EDGE ( 'NONE', *, *, #5989, .T. ) ;
#18331=FACE_OUTER_BOUND ( 'NONE', #68, .T. ) ;
#18332=LINE ( 'NONE', #24222, #7083 ) ;
#18351=DIRECTION ( 'NONE',  ( -1.000000000000000000, -2.999999999999999839E-15, 0.000000000000000000 ) ) ;
#18365=DIRECTION ( 'NONE',  ( 1.327674326049719602E-15, -0.4425581086832399147, 0.8967398287344627850 ) ) ;
#18382=ORIENTED_EDGE ( 'NONE', *, *, #24899, .F. ) ;
#18383=VERTEX_POINT ( 'NONE', #3561 ) ;
#18389=VECTOR ( 'NONE', #8148, 1000.000000000000000 ) ;
#18399=EDGE_CURVE ( 'NONE', #13201, #4779, #5633, .T. ) ;
#18407=AXIS2_PLACEMENT_3D ( 'NONE', #451, #16049, #15921 ) ;
#18411=AXIS2_PLACEMENT_3D ( 'NONE', #24549, #2918, #6672 ) ;
#18425=LINE ( 'NONE', #12518, #24600 ) ;
#18448=ORIENTED_EDGE ( 'NONE', *, *, #8636, .F. ) ;
#18450=VERTEX_POINT ( 'NONE', #7315 ) ;
#18461=CARTESIAN_POINT ( 'NONE',  ( 42.96606138205697789, -5.898435835062210586, -2.003809078978638247 ) ) ;
#18463=CIRCLE ( 'NONE', #8191, 1.000000000000012657 ) ;
#18473=CARTESIAN_POINT ( 'NONE',  ( 33.66606138205694521, 5.208890205473720059, 5.429380561359602453 ) ) ;
#18480=VERTEX_POINT ( 'NONE', #5383 ) ;
#18492=EDGE_LOOP ( 'NONE', ( #1620, #4193, #10437, #9155 ) ) ;
#18495=VECTOR ( 'NONE', #1757, 1000.000000000000000 ) ;
#18496=DIRECTION ( 'NONE',  ( 1.734723475976807094E-15, -0.7516416929448819229, -0.6595716529892350355 ) ) ;
#18506=VECTOR ( 'NONE', #25161, 1000.000000000000000 ) ;
#18509=VECTOR ( 'NONE', #11760, 1000.000000000000000 ) ;
#18517=ORIENTED_EDGE ( 'NONE', *, *, #20605, .T. ) ;
#18529=EDGE_CURVE ( 'NONE', #17733, #9987, #21478, .T. ) ;
#18566=CARTESIAN_POINT ( 'NONE',  ( 36.06606138205694378, 4.312150376739267266, 4.986822452676363149 ) ) ;
#18577=ORIENTED_EDGE ( 'NONE', *, *, #8964, .F. ) ;
#18584=DIRECTION ( 'NONE',  ( -1.734723475976807292E-15, 0.7516416929448820339, 0.6595716529892350355 ) ) ;
#18597=VERTEX_POINT ( 'NONE', #10269 ) ;
#18606=ORIENTED_EDGE ( 'NONE', *, *, #7665, .F. ) ;
#18609=ORIENTED_EDGE ( 'NONE', *, *, #9283, .F. ) ;
#18610=DIRECTION ( 'NONE',  ( -1.327674326049719602E-15, 0.4425581086832399147, -0.8967398287344627850 ) ) ;
#18619=ORIENTED_EDGE ( 'NONE', *, *, #15799, .F. ) ;
#18630=VECTOR ( 'NONE', #1976, 1000.000000000000000 ) ;
#18631=CYLINDRICAL_SURFACE ( 'NONE', #9050, 1.000000000000012657 ) ;
#18638=FACE_OUTER_BOUND ( 'NONE', #15824, .T. ) ;
#18642=CIRCLE ( 'NONE', #10012, 1.000000000000000888 ) ;
#18652=DIRECTION ( 'NONE',  ( -1.225631768639319301E-15, 0.4425581086832399147, -0.8967398287344627850 ) ) ;
#18656=PLANE ( 'NONE',  #4221 ) ;
#18658=VECTOR ( 'NONE', #20941, 1000.000000000000000 ) ;
#18662=ORIENTED_EDGE ( 'NONE', *, *, #16079, .F. ) ;
#18664=DIRECTION ( 'NONE',  ( -4.625929269271484533E-15, 0.8967398287344634511, 0.4425581086832385824 ) ) ;
#18665=ORIENTED_EDGE ( 'NONE', *, *, #12929, .F. ) ;
#18666=EDGE_LOOP ( 'NONE', ( #5195, #6641, #23977, #24220 ) ) ;
#18669=AXIS2_PLACEMENT_3D ( 'NONE', #22795, #3204, #1278 ) ;
#18672=EDGE_CURVE ( 'NONE', #18480, #9092, #2014, .T. ) ;
#18680=ORIENTED_EDGE ( 'NONE', *, *, #16350, .F. ) ;
#18694=VERTEX_POINT ( 'NONE', #18133 ) ;
#18695=CARTESIAN_POINT ( 'NONE',  ( 42.96606138205694947, 3.409598742320834930, 3.426245460917042074 ) ) ;
#18708=EDGE_CURVE ( 'NONE', #1835, #18383, #15146, .T. ) ;
#18713=EDGE_CURVE ( 'NONE', #12829, #18144, #19932, .T. ) ;
#18737=FACE_BOUND ( 'NONE', #25463, .T. ) ;
#18742=CARTESIAN_POINT ( 'NONE',  ( 37.31606138205702194, -21.82181003913286688, 31.95585308007612468 ) ) ;
#18747=VECTOR ( 'NONE', #7854, 1000.000000000000000 ) ;
#18753=CARTESIAN_POINT ( 'NONE',  ( 45.81606138205707168, -37.70325315460877391, 65.37863370302704880 ) ) ;
#18760=DIRECTION ( 'NONE',  ( 3.469446951953570407E-15, -0.8967398287344626739, -0.4425581086832399702 ) ) ;
#18766=ORIENTED_EDGE ( 'NONE', *, *, #6723, .T. ) ;
#18767=PLANE ( 'NONE',  #6663 ) ;
#18790=LINE ( 'NONE', #2805, #9911 ) ;
#18799=CARTESIAN_POINT ( 'NONE',  ( 45.81606138205706458, -35.90867894478441968, 74.07034463014319670 ) ) ;
#18813=CARTESIAN_POINT ( 'NONE',  ( 33.66606138205698073, -6.570990706613086374, -2.335727660491067503 ) ) ;
#18820=DIRECTION ( 'NONE',  ( -1.327674326049709741E-15, 0.4425581086832367506, -0.8967398287344643393 ) ) ;
#18821=AXIS2_PLACEMENT_3D ( 'NONE', #18062, #2073, #18318 ) ;
#18822=VECTOR ( 'NONE', #19779, 1000.000000000000000 ) ;
#18826=ORIENTED_EDGE ( 'NONE', *, *, #509, .F. ) ;
#18827=LINE ( 'NONE', #22939, #18131 ) ;
#18829=ORIENTED_EDGE ( 'NONE', *, *, #594, .T. ) ;
#18831=PLANE ( 'NONE',  #11736 ) ;
#18860=ORIENTED_EDGE ( 'NONE', *, *, #2586, .F. ) ;
#18861=DIRECTION ( 'NONE',  ( 1.000000000000000000, 2.740734061208483951E-15, -1.279526567694519919E-16 ) ) ;
#18862=CARTESIAN_POINT ( 'NONE',  ( 29.81606138205697931, -5.918777154956199382, -5.916875169744970187 ) ) ;
#18867=CARTESIAN_POINT ( 'NONE',  ( 34.81606138205696510, -1.975699482566735776, -4.057200616784870206 ) ) ;
#18870=EDGE_CURVE ( 'NONE', #15010, #15653, #17625, .T. ) ;
#18876=DIRECTION ( 'NONE',  ( 1.271715504244016160E-15, -0.4425581086832399147, 0.8967398287344627850 ) ) ;
#18892=CIRCLE ( 'NONE', #7788, 1.750000000000001554 ) ;
#18895=ORIENTED_EDGE ( 'NONE', *, *, #23462, .F. ) ;
#18906=DIRECTION ( 'NONE',  ( 2.690219486203388234E-15, -0.8967398287344627850, -0.4425581086832399147 ) ) ;
#18909=DIRECTION ( 'NONE',  ( 1.327674326049719602E-15, -0.4425581086832399147, 0.8967398287344627850 ) ) ;
#18915=CARTESIAN_POINT ( 'NONE',  ( 40.56606138205697931, -5.948051402551118194, 9.959574150503843981 ) ) ;
#18920=CARTESIAN_POINT ( 'NONE',  ( 30.81606138205697221, -3.542416608809866752, -4.744096181734387407 ) ) ;
#18956=DIRECTION ( 'NONE',  ( 1.000000000000000000, 2.999999999999999839E-15, 0.000000000000000000 ) ) ;
#18965=ORIENTED_EDGE ( 'NONE', *, *, #8973, .T. ) ;
#18975=ORIENTED_EDGE ( 'NONE', *, *, #14621, .T. ) ;
#18977=DIRECTION ( 'NONE',  ( -1.327674326049719602E-15, 0.4425581086832399147, -0.8967398287344627850 ) ) ;
#18984=VECTOR ( 'NONE', #11015, 1000.000000000000000 ) ;
#18997=DIRECTION ( 'NONE',  ( 1.000000000000000000, 2.999999999999999839E-15, 0.000000000000000000 ) ) ;
#19017=EDGE_CURVE ( 'NONE', #13333, #18144, #15042, .T. ) ;
#19022=LINE ( 'NONE', #24287, #21030 ) ;
#19023=EDGE_LOOP ( 'NONE', ( #11927, #2932, #17484, #22103 ) ) ;
#19039=VERTEX_POINT ( 'NONE', #2923 ) ;
#19040=PLANE ( 'NONE',  #21111 ) ;
#19057=EDGE_CURVE ( 'NONE', #15655, #8846, #6339, .T. ) ;
#19059=DIRECTION ( 'NONE',  ( -2.480932259201170508E-15, 0.9193606199277819524, 0.3934158747763039088 ) ) ;
#19061=ORIENTED_EDGE ( 'NONE', *, *, #25294, .F. ) ;
#19077=ORIENTED_EDGE ( 'NONE', *, *, #14606, .F. ) ;
#19081=ORIENTED_EDGE ( 'NONE', *, *, #23270, .T. ) ;
#19083=EDGE_CURVE ( 'NONE', #14416, #10854, #4404, .T. ) ;
#19090=ORIENTED_EDGE ( 'NONE', *, *, #12633, .T. ) ;
#19094=FILL_AREA_STYLE ('',( #13544 ) ) ;
#19097=CARTESIAN_POINT ( 'NONE',  ( 35.56606138205700063, -13.51824891481310509, 37.72654391001022134 ) ) ;
#19099=VECTOR ( 'NONE', #2722, 1000.000000000000000 ) ;
#19106=DIRECTION ( 'NONE',  ( 1.000000000000000000, 2.999999999999999839E-15, 0.000000000000000000 ) ) ;
#19108=DIRECTION ( 'NONE',  ( -2.048868001712898319E-15, 0.6595716529892350355, -0.7516416929448821449 ) ) ;
#19114=VECTOR ( 'NONE', #13334, 1000.000000000000000 ) ;
#19120=ORIENTED_EDGE ( 'NONE', *, *, #14483, .T. ) ;
#19121=CARTESIAN_POINT ( 'NONE',  ( 30.81606138205696865, -3.028410647649177889, 0.3252050635115383281 ) ) ;
#19125=ORIENTED_EDGE ( 'NONE', *, *, #8624, .T. ) ;
#19127=DIRECTION ( 'NONE',  ( -1.000000000000000000, -2.999999999999999839E-15, 0.000000000000000000 ) ) ;
#19128=FACE_OUTER_BOUND ( 'NONE', #22244, .T. ) ;
#19130=LINE ( 'NONE', #8966, #16621 ) ;
#19145=DIRECTION ( 'NONE',  ( -1.000000000000000000, -2.602085213965208275E-15, 0.000000000000000000 ) ) ;
#19148=ORIENTED_EDGE ( 'NONE', *, *, #11549, .F. ) ;
#19161=ORIENTED_EDGE ( 'NONE', *, *, #714, .F. ) ;
#19164=LINE ( 'NONE', #23526, #498 ) ;
#19167=PRODUCT ( 'Upper Metal Lever Arm', 'Upper Metal Lever Arm', '', ( #3757 ) ) ;
#19173=DIRECTION ( 'NONE',  ( 2.942087424212892849E-15, -0.8967398287344627850, -0.4425581086832399147 ) ) ;
#19178=EDGE_CURVE ( 'NONE', #8257, #1835, #1885, .T. ) ;
#19180=FACE_OUTER_BOUND ( 'NONE', #19023, .T. ) ;
#19183=ORIENTED_EDGE ( 'NONE', *, *, #19568, .T. ) ;
#19197=EDGE_LOOP ( 'NONE', ( #13663, #6764, #4325, #16161 ) ) ;
#19201=ORIENTED_EDGE ( 'NONE', *, *, #25294, .T. ) ;
#19207=AXIS2_PLACEMENT_3D ( 'NONE', #20813, #11020, #22985 ) ;
#19226=AXIS2_PLACEMENT_3D ( 'NONE', #9138, #20586, #22392 ) ;
#19240=LINE ( 'NONE', #5977, #14936 ) ;
#19246=VECTOR ( 'NONE', #9765, 1000.000000000000000 ) ;
#19251=ORIENTED_EDGE ( 'NONE', *, *, #21706, .F. ) ;
#19266=EDGE_CURVE ( 'NONE', #17666, #14180, #3452, .T. ) ;
#19267=PLANE ( 'NONE',  #2089 ) ;
#19275=CARTESIAN_POINT ( 'NONE',  ( 40.71606138205696368, -0.07962245140794542431, -2.393377716359348817 ) ) ;
#19277=LINE ( 'NONE', #11316, #6618 ) ;
#19303=CARTESIAN_POINT ( 'NONE',  ( 29.81606138205694734, 5.290470704224588872, -0.3848988112044732235 ) ) ;
#19308=VECTOR ( 'NONE', #18652, 1000.000000000000000 ) ;
#19311=EDGE_CURVE ( 'NONE', #19523, #16500, #22976, .T. ) ;
#19321=ORIENTED_EDGE ( 'NONE', *, *, #7228, .T. ) ;
#19335=APPLICATION_CONTEXT ( 'automotive_design' ) ;
#19349=EDGE_CURVE ( 'NONE', #3431, #13994, #14140, .T. ) ;
#19365=AXIS2_PLACEMENT_3D ( 'NONE', #24531, #6789, #2772 ) ;
#19371=LINE ( 'NONE', #17702, #1361 ) ;
#19373=DIRECTION ( 'NONE',  ( 1.000000000000000000, 2.973811673103095397E-15, 0.000000000000000000 ) ) ;
#19384=EDGE_LOOP ( 'NONE', ( #22668, #20615, #13076, #16194 ) ) ;
#19385=CARTESIAN_POINT ( 'NONE',  ( 40.31606138205701484, -19.58709462196289763, 24.03834292329984379 ) ) ;
#19399=EDGE_CURVE ( 'NONE', #58, #7231, #8344, .T. ) ;
#19403=VERTEX_POINT ( 'NONE', #16186 ) ;
#19414=VECTOR ( 'NONE', #23677, 1000.000000000000000 ) ;
#19416=ORIENTED_EDGE ( 'NONE', *, *, #14064, .F. ) ;
#19419=ORIENTED_EDGE ( 'NONE', *, *, #391, .F. ) ;
#19433=DIRECTION ( 'NONE',  ( 0.000000000000000000, -0.4425581086832400257, 0.8967398287344627850 ) ) ;
#19434=ADVANCED_FACE ( 'NONE', ( #19675 ), #2270, .F. ) ;
#19435=VECTOR ( 'NONE', #20301, 1000.000000000000114 ) ;
#19453=AXIS2_PLACEMENT_3D ( 'NONE', #13209, #3142, #12705 ) ;
#19483=MECHANICAL_DESIGN_GEOMETRIC_PRESENTATION_REPRESENTATION('',(#5123),#552);
#19484=EDGE_CURVE ( 'NONE', #559, #786, #6525, .T. ) ;
#19496=VECTOR ( 'NONE', #22547, 1000.000000000000000 ) ;
#19507=DIRECTION ( 'NONE',  ( 1.000000000000000000, 2.999999999999999839E-15, 0.000000000000000000 ) ) ;
#19521=DIRECTION ( 'NONE',  ( 1.734723475976805517E-15, -0.4425581086832399702, 0.8967398287344627850 ) ) ;
#19523=VERTEX_POINT ( 'NONE', #10531 ) ;
#19524=DIRECTION ( 'NONE',  ( -2.163881430871171154E-15, 0.7573960774932753104, -0.6529557272876933549 ) ) ;
#19541=ORIENTED_EDGE ( 'NONE', *, *, #18529, .F. ) ;
#19553=VERTEX_POINT ( 'NONE', #8854 ) ;
#19556=EDGE_LOOP ( 'NONE', ( #19785, #12070, #4785, #3166 ) ) ;
#19568=EDGE_CURVE ( 'NONE', #6874, #5497, #11029, .T. ) ;
#19572=DIRECTION ( 'NONE',  ( -1.000000000000000000, -2.999999999999999839E-15, 0.000000000000000000 ) ) ;
#19587=LINE ( 'NONE', #5556, #11962 ) ;
#19591=CARTESIAN_POINT ( 'NONE',  ( 30.81606138205697931, -5.918777154956195830, -5.916875169744970187 ) ) ;
#19592=CARTESIAN_POINT ( 'NONE',  ( 46.81606138205697221, -4.349482454670835274, -5.142398479549302515 ) ) ;
#19597=DIRECTION ( 'NONE',  ( -1.000000000000000000, -2.967680473743455856E-15, -2.960622826238914985E-16 ) ) ;
#19598=LINE ( 'NONE', #1939, #8517 ) ;
#19616=ORIENTED_EDGE ( 'NONE', *, *, #14158, .F. ) ;
#19624=AXIS2_PLACEMENT_3D ( 'NONE', #5954, #11763, #25117 ) ;
#19625=ORIENTED_EDGE ( 'NONE', *, *, #20830, .T. ) ;
#19629=VECTOR ( 'NONE', #9083, 1000.000000000000000 ) ;
#19637=ADVANCED_FACE ( 'NONE', ( #3664 ), #15269, .F. ) ;
#19640=DIRECTION ( 'NONE',  ( 2.412663730047098310E-15, -0.8967398287344625629, -0.4425581086832404143 ) ) ;
#19643=ORIENTED_EDGE ( 'NONE', *, *, #10742, .F. ) ;
#19645=CARTESIAN_POINT ( 'NONE',  ( 31.56606138205708589, -42.63947656429714783, 70.74856838136764736 ) ) ;
#19650=CARTESIAN_POINT ( 'NONE',  ( 33.66606138205698073, -7.467730535347549825, -2.778285769174305919 ) ) ;
#19656=VERTEX_POINT ( 'NONE', #7422 ) ;
#19660=FACE_OUTER_BOUND ( 'NONE', #15119, .T. ) ;
#19675=FACE_OUTER_BOUND ( 'NONE', #17327, .T. ) ;
#19677=CARTESIAN_POINT ( 'NONE',  ( 34.81606138205696510, -1.975699482566735776, -4.057200616784870206 ) ) ;
#19680=ORIENTED_EDGE ( 'NONE', *, *, #19349, .T. ) ;
#19693=AXIS2_PLACEMENT_3D ( 'NONE', #6308, #21634, #10048 ) ;
#19724=LINE ( 'NONE', #17418, #10361 ) ;
#19743=VERTEX_POINT ( 'NONE', #19385 ) ;
#19745=DIRECTION ( 'NONE',  ( 1.327674326049719602E-15, -0.4425581086832399147, 0.8967398287344627850 ) ) ;
#19749=VECTOR ( 'NONE', #655, 1000.000000000000000 ) ;
#19750=ORIENTED_EDGE ( 'NONE', *, *, #11473, .T. ) ;
#19758=FACE_OUTER_BOUND ( 'NONE', #14797, .T. ) ;
#19759=ORIENTED_EDGE ( 'NONE', *, *, #24429, .T. ) ;
#19779=DIRECTION ( 'NONE',  ( 1.000000000000000000, 2.999999999999999839E-15, 0.000000000000000000 ) ) ;
#19785=ORIENTED_EDGE ( 'NONE', *, *, #4532, .T. ) ;
#19801=EDGE_CURVE ( 'NONE', #15157, #13632, #15516, .T. ) ;
#19808=CARTESIAN_POINT ( 'NONE',  ( 29.81606138205706458, -34.55876147768187678, 70.30501292735635843 ) ) ;
#19815=EDGE_CURVE ( 'NONE', #15268, #8846, #17089, .T. ) ;
#19823=DIRECTION ( 'NONE',  ( 1.000000000000000000, 2.751104698760144965E-15, -1.228345504986737969E-16 ) ) ;
#19829=CARTESIAN_POINT ( 'NONE',  ( 35.56606138205703616, -24.72749677399389157, 32.19456755146972426 ) ) ;
#19832=CARTESIAN_POINT ( 'NONE',  ( 34.81606138205696510, -1.316127829577488528, -4.808842309729777220 ) ) ;
#19836=DIRECTION ( 'NONE',  ( -2.412663730047099099E-15, 0.8967398287344627850, 0.4425581086832399147 ) ) ;
#19867=ADVANCED_FACE ( 'NONE', ( #2487 ), #424, .T. ) ;
#19875=EDGE_LOOP ( 'NONE', ( #1778, #6143, #5089, #21623 ) ) ;
#19877=ORIENTED_EDGE ( 'NONE', *, *, #6858, .T. ) ;
#19879=CARTESIAN_POINT ( 'NONE',  ( 33.80827534892208064, -20.02093502212017029, 26.61211107664843212 ) ) ;
#19882=ORIENTED_EDGE ( 'NONE', *, *, #17366, .T. ) ;
#19893=ORIENTED_EDGE ( 'NONE', *, *, #7052, .F. ) ;
#19894=ORIENTED_EDGE ( 'NONE', *, *, #15336, .T. ) ;
#19895=LINE ( 'NONE', #2234, #6326 ) ;
#19900=CARTESIAN_POINT ( 'NONE',  ( 29.81606138205707524, -38.13418765192407989, 68.51141129791366780 ) ) ;
#19901=EDGE_LOOP ( 'NONE', ( #4107, #13411 ) ) ;
#19903=AXIS2_PLACEMENT_3D ( 'NONE', #1527, #13404, #13282 ) ;
#19929=ORIENTED_EDGE ( 'NONE', *, *, #4044, .T. ) ;
#19930=DIRECTION ( 'NONE',  ( 1.327674326049719602E-15, -0.4425581086832399147, 0.8967398287344627850 ) ) ;
#19932=LINE ( 'NONE', #459, #19246 ) ;
#19937=DIRECTION ( 'NONE',  ( 1.000000000000000000, 2.554104467024131702E-15, 1.134076704137112863E-15 ) ) ;
#19941=ORIENTED_EDGE ( 'NONE', *, *, #8500, .F. ) ;
#19963=ADVANCED_FACE ( 'NONE', ( #23999 ), #25417, .T. ) ;
#19976=VECTOR ( 'NONE', #21627, 1000.000000000000000 ) ;
#19981=CARTESIAN_POINT ( 'NONE',  ( 36.06606138205697931, -5.948051402551132405, 9.959574150503843981 ) ) ;
#20000=CARTESIAN_POINT ( 'NONE',  ( 30.81606138205696510, -0.7562224151693580643, -1.633662118351544734 ) ) ;
#20015=ORIENTED_EDGE ( 'NONE', *, *, #15109, .F. ) ;
#20024=DIRECTION ( 'NONE',  ( 2.792262043613788535E-15, -0.8967398287344627850, -0.4425581086832399147 ) ) ;
#20031=LINE ( 'NONE', #10248, #23434 ) ;
#20032=CARTESIAN_POINT ( 'NONE',  ( 29.81606138205696155, -0.7562224151693598406, -1.633662118351544734 ) ) ;
#20035=VERTEX_POINT ( 'NONE', #10751 ) ;
#20036=ORIENTED_EDGE ( 'NONE', *, *, #8636, .T. ) ;
#20069=ORIENTED_EDGE ( 'NONE', *, *, #24177, .F. ) ;
#20075=CARTESIAN_POINT ( 'NONE',  ( 41.06606138205703616, -24.72749677399387735, 32.19456755146972426 ) ) ;
#20089=EDGE_LOOP ( 'NONE', ( #14828, #16959, #19643, #14392 ) ) ;
#20112=VECTOR ( 'NONE', #9740, 1000.000000000000000 ) ;
#20115=CARTESIAN_POINT ( 'NONE',  ( 45.81606138205705037, -30.46100403034031245, 72.05704881431053366 ) ) ;
#20122=DIRECTION ( 'NONE',  ( -1.000000000000000000, -3.091505625455828697E-15, -4.515976121274772923E-17 ) ) ;
#20131=VECTOR ( 'NONE', #6344, 1000.000000000000000 ) ;
#20135=LINE ( 'NONE', #16005, #3428 ) ;
#20146=DIRECTION ( 'NONE',  ( 2.341661252633485168E-15, -0.7516416929448815898, -0.6595716529892353686 ) ) ;
#20153=LINE ( 'NONE', #11802, #11966 ) ;
#20162=DIRECTION ( 'NONE',  ( 0.000000000000000000, 0.4425581086832397482, -0.8967398287344628960 ) ) ;
#20166=VERTEX_POINT ( 'NONE', #20527 ) ;
#20179=VECTOR ( 'NONE', #22276, 1000.000000000000000 ) ;
#20183=DIRECTION ( 'NONE',  ( 1.000000000000000000, 3.066740595113354287E-15, 9.534026549497653239E-17 ) ) ;
#20186=DIRECTION ( 'NONE',  ( -2.442401846778130416E-15, 0.8967398287344627850, 0.4425581086832399147 ) ) ;
#20187=EDGE_CURVE ( 'NONE', #13086, #10846, #14478, .T. ) ;
#20188=DIRECTION ( 'NONE',  ( -2.048868001712896742E-15, 0.6595716529892345914, -0.7516416929448823669 ) ) ;
#20199=ORIENTED_EDGE ( 'NONE', *, *, #23489, .F. ) ;
#20218=ORIENTED_EDGE ( 'NONE', *, *, #18672, .F. ) ;
#20223=DIRECTION ( 'NONE',  ( 1.000000000000000000, 2.751104698760144965E-15, -1.228345504986737969E-16 ) ) ;
#20225=VERTEX_POINT ( 'NONE', #17058 ) ;
#20230=AXIS2_PLACEMENT_3D ( 'NONE', #4362, #6295, #16576 ) ;
#20241=ORIENTED_EDGE ( 'NONE', *, *, #6176, .F. ) ;
#20243=AXIS2_PLACEMENT_3D ( 'NONE', #17613, #25317, #25443 ) ;
#20250=ORIENTED_EDGE ( 'NONE', *, *, #23549, .F. ) ;
#20254=FACE_OUTER_BOUND ( 'NONE', #15277, .T. ) ;
#20277=VERTEX_POINT ( 'NONE', #3630 ) ;
#20280=AXIS2_PLACEMENT_3D ( 'NONE', #6644, #16689, #4839 ) ;
#20287=VERTEX_POINT ( 'NONE', #20916 ) ;
#20301=DIRECTION ( 'NONE',  ( -2.048868001712899108E-15, 0.6595716529892353686, -0.7516416929448815898 ) ) ;
#20303=CARTESIAN_POINT ( 'NONE',  ( 31.56606138205697576, -5.918777154956194053, -5.916875169744970187 ) ) ;
#20312=LINE ( 'NONE', #22736, #2172 ) ;
#20320=DIRECTION ( 'NONE',  ( 1.123589211228918605E-15, -0.4425581086832399147, 0.8967398287344627850 ) ) ;
#20321=CYLINDRICAL_SURFACE ( 'NONE', #22956, 1.500000000000000222 ) ;
#20334=CIRCLE ( 'NONE', #19903, 1.750000000000000222 ) ;
#20339=FACE_OUTER_BOUND ( 'NONE', #1571, .T. ) ;
#20368=CARTESIAN_POINT ( 'NONE',  ( 30.81606138205696510, -0.7562224151693580643, -1.633662118351544734 ) ) ;
#20374=VERTEX_POINT ( 'NONE', #13065 ) ;
#20401=EDGE_CURVE ( 'NONE', #24942, #17659, #2077, .T. ) ;
#20407=VERTEX_POINT ( 'NONE', #8145 ) ;
#20413=ORIENTED_EDGE ( 'NONE', *, *, #19057, .F. ) ;
#20415=FACE_OUTER_BOUND ( 'NONE', #10432, .T. ) ;
#20417=ORIENTED_EDGE ( 'NONE', *, *, #6176, .T. ) ;
#20422=EDGE_CURVE ( 'NONE', #11230, #19656, #9708, .T. ) ;
#20425=EDGE_LOOP ( 'NONE', ( #6219, #11561, #13635, #11546, #20250, #21313 ) ) ;
#20440=ORIENTED_EDGE ( 'NONE', *, *, #7858, .T. ) ;
#20449=EDGE_CURVE ( 'NONE', #20703, #24865, #9831, .T. ) ;
#20464=DIRECTION ( 'NONE',  ( -1.327674326049719602E-15, 0.4425581086832399147, -0.8967398287344627850 ) ) ;
#20489=DIRECTION ( 'NONE',  ( -1.000000000000000000, -2.999999999999999839E-15, 0.000000000000000000 ) ) ;
#20497=EDGE_LOOP ( 'NONE', ( #4295, #11068, #15274, #11038, #2709, #13639 ) ) ;
#20498=EDGE_CURVE ( 'NONE', #9852, #20804, #4157, .T. ) ;
#20500=LINE ( 'NONE', #14825, #15508 ) ;
#20512=FACE_OUTER_BOUND ( 'NONE', #9462, .T. ) ;
#20519=EDGE_CURVE ( 'NONE', #12687, #13086, #21668, .T. ) ;
#20527=CARTESIAN_POINT ( 'NONE',  ( 29.81606138205697576, -4.349482454670887677, -5.142398479549302515 ) ) ;
#20528=CIRCLE ( 'NONE', #24622, 1.000000000000000888 ) ;
#20536=ORIENTED_EDGE ( 'NONE', *, *, #10660, .T. ) ;
#20542=ORIENTED_EDGE ( 'NONE', *, *, #17368, .T. ) ;
#20568=FACE_OUTER_BOUND ( 'NONE', #21331, .T. ) ;
#20573=ADVANCED_FACE ( 'NONE', ( #2453 ), #24212, .F. ) ;
#20581=EDGE_CURVE ( 'NONE', #7686, #18144, #16752, .T. ) ;
#20586=DIRECTION ( 'NONE',  ( -2.792262043613788535E-15, 0.8967398287344627850, 0.4425581086832399147 ) ) ;
#20590=CARTESIAN_POINT ( 'NONE',  ( 42.96606138205698500, -7.467730535347522292, -2.778285769174305919 ) ) ;
#20593=VERTEX_POINT ( 'NONE', #14569 ) ;
#20600=VERTEX_POINT ( 'NONE', #24589 ) ;
#20605=EDGE_CURVE ( 'NONE', #7382, #23154, #1029, .T. ) ;
#20615=ORIENTED_EDGE ( 'NONE', *, *, #21451, .F. ) ;
#20623=CARTESIAN_POINT ( 'NONE',  ( 29.81606138205696155, -0.2703287878658162113, 1.505452687840413972 ) ) ;
#20630=DIRECTION ( 'NONE',  ( -2.792262043613788535E-15, 0.8967398287344627850, 0.4425581086832399147 ) ) ;
#20672=ORIENTED_EDGE ( 'NONE', *, *, #8684, .T. ) ;
#20678=VECTOR ( 'NONE', #8748, 1000.000000000000000 ) ;
#20684=EDGE_CURVE ( 'NONE', #24942, #12724, #2823, .T. ) ;
#20686=ADVANCED_FACE ( 'NONE', ( #16245 ), #6463, .F. ) ;
#20691=DIRECTION ( 'NONE',  ( 1.000000000000000000, 2.999999999999999839E-15, 0.000000000000000000 ) ) ;
#20703=VERTEX_POINT ( 'NONE', #18566 ) ;
#20707=ORIENTED_EDGE ( 'NONE', *, *, #16759, .T. ) ;
#20709=ORIENTED_EDGE ( 'NONE', *, *, #4430, .T. ) ;
#20710=DIRECTION ( 'NONE',  ( 2.602085213965210642E-15, -0.8967398287344635621, -0.4425581086832386379 ) ) ;
#20722=CARTESIAN_POINT ( 'NONE',  ( 43.31606138205697221, -5.022037326221694187, -5.474317061061731771 ) ) ;
#20734=AXIS2_PLACEMENT_3D ( 'NONE', #7092, #23296, #7473 ) ;
#20739=DIRECTION ( 'NONE',  ( 1.327674326049719602E-15, -0.4425581086832399147, 0.8967398287344627850 ) ) ;
#20742=CARTESIAN_POINT ( 'NONE',  ( 45.81606138205695800, -0.7562224151693129892, -1.633662118351544734 ) ) ;
#20784=DIRECTION ( 'NONE',  ( 1.000000000000000000, 2.999999999999999839E-15, 0.000000000000000000 ) ) ;
#20804=VERTEX_POINT ( 'NONE', #11096 ) ;
#20813=CARTESIAN_POINT ( 'NONE',  ( 31.91606138205695231, 3.586515973360766996, -0.5067327973472466329 ) ) ;
#20830=EDGE_CURVE ( 'NONE', #20166, #24103, #15199, .T. ) ;
#20837=CARTESIAN_POINT ( 'NONE',  ( 36.31606138205698642, -9.092667827980706718, 28.75914562266559926 ) ) ;
#20853=FACE_OUTER_BOUND ( 'NONE', #6684, .T. ) ;
#20876=DIRECTION ( 'NONE',  ( 1.000000000000000000, 3.194449454093636459E-15, 9.596449257708877207E-17 ) ) ;
#20885=DIRECTION ( 'NONE',  ( -2.312964634635742267E-15, 0.8967398287344626739, 0.4425581086832399147 ) ) ;
#20897=VERTEX_POINT ( 'NONE', #18041 ) ;
#20916=CARTESIAN_POINT ( 'NONE',  ( 45.81606138205695800, -0.7562224151693129892, -1.633662118351544734 ) ) ;
#20920=ORIENTED_EDGE ( 'NONE', *, *, #4866, .F. ) ;
#20926=EDGE_CURVE ( 'NONE', #2906, #15674, #6187, .T. ) ;
#20931=FACE_OUTER_BOUND ( 'NONE', #1017, .T. ) ;
#20932=CARTESIAN_POINT ( 'NONE',  ( 38.31606138205697931, -6.672912525257896021, -0.4345143786933236552 ) ) ;
#20941=DIRECTION ( 'NONE',  ( -2.792262043613788535E-15, 0.8967398287344627850, 0.4425581086832399147 ) ) ;
#20968=VECTOR ( 'NONE', #1824, 1000.000000000000000 ) ;
#20985=CARTESIAN_POINT ( 'NONE',  ( 41.06606138205698642, -9.092667827980692508, 28.75914562266559926 ) ) ;
#20990=ADVANCED_FACE ( 'NONE', ( #8116 ), #9800, .F. ) ;
#20996=DIRECTION ( 'NONE',  ( 1.047880217021202589E-15, -0.4425581086832399147, 0.8967398287344627850 ) ) ;
#21011=LINE ( 'NONE', #2862, #8232 ) ;
#21030=VECTOR ( 'NONE', #6652, 1000.000000000000000 ) ;
#21034=CARTESIAN_POINT ( 'NONE',  ( 35.91606138205695942, 0.5799492015812600654, -3.145019409304214530 ) ) ;
#21052=ORIENTED_EDGE ( 'NONE', *, *, #25469, .F. ) ;
#21054=CARTESIAN_POINT ( 'NONE',  ( 40.31606138205701484, -19.40517585842702175, 23.66972737280834238 ) ) ;
#21057=ORIENTED_EDGE ( 'NONE', *, *, #23142, .F. ) ;
#21064=CARTESIAN_POINT ( 'NONE',  ( 35.91606138205695942, -0.07962245140795930209, -2.393377716359348817 ) ) ;
#21080=CARTESIAN_POINT ( 'NONE',  ( 30.81606138205706813, -35.90387122078356441, 69.64117576433150703 ) ) ;
#21083=PLANE ( 'NONE',  #4167 ) ;
#21092=VECTOR ( 'NONE', #8582, 1000.000000000000000 ) ;
#21094=CARTESIAN_POINT ( 'NONE',  ( 40.31606138205701484, -20.02093502212014897, 26.61211107664843212 ) ) ;
#21104=DIRECTION ( 'NONE',  ( -2.048868001712899108E-15, 0.6595716529892353686, -0.7516416929448815898 ) ) ;
#21109=ORIENTED_EDGE ( 'NONE', *, *, #24744, .T. ) ;
#21111=AXIS2_PLACEMENT_3D ( 'NONE', #17619, #9645, #5892 ) ;
#21121=ORIENTED_EDGE ( 'NONE', *, *, #20422, .F. ) ;
#21132=AXIS2_PLACEMENT_3D ( 'NONE', #3987, #16084, #13657 ) ;
#21138=CIRCLE ( 'NONE', #5493, 1.000000000000000000 ) ;
#21154=FACE_OUTER_BOUND ( 'NONE', #11180, .T. ) ;
#21156=AXIS2_PLACEMENT_3D ( 'NONE', #10125, #14242, #16282 ) ;
#21158=LINE ( 'NONE', #21658, #5007 ) ;
#21160=DIRECTION ( 'NONE',  ( 2.011972697750610993E-15, -0.6595716529892349245, 0.7516416929448819229 ) ) ;
#21161=AXIS2_PLACEMENT_3D ( 'NONE', #8458, #4716, #24397 ) ;
#21162=DIRECTION ( 'NONE',  ( 3.469446951953614189E-15, -0.8967398287344635621, -0.4425581086832386379 ) ) ;
#21187=EDGE_LOOP ( 'NONE', ( #4261, #3978, #8828, #14153 ) ) ;
#21190=CARTESIAN_POINT ( 'NONE',  ( 29.81606138205707524, -38.13418765192407989, 68.51141129791366780 ) ) ;
#21193=ORIENTED_EDGE ( 'NONE', *, *, #14064, .T. ) ;
#21202=PLANE ( 'NONE',  #7706 ) ;
#21208=FACE_OUTER_BOUND ( 'NONE', #20089, .T. ) ;
#21214=DIRECTION ( 'NONE',  ( -1.327674326049719602E-15, 0.4425581086832399147, -0.8967398287344627850 ) ) ;
#21215=VERTEX_POINT ( 'NONE', #21233 ) ;
#21230=DIRECTION ( 'NONE',  ( -1.327674326049719602E-15, 0.4425581086832399147, -0.8967398287344627850 ) ) ;
#21232=VERTEX_POINT ( 'NONE', #12876 ) ;
#21233=CARTESIAN_POINT ( 'NONE',  ( 40.31606138205702194, -21.37925193044962313, 31.05911325134166034 ) ) ;
#21244=DIRECTION ( 'NONE',  ( 1.327674326049719602E-15, -0.4425581086832399147, 0.8967398287344627850 ) ) ;
#21248=CARTESIAN_POINT ( 'NONE',  ( 45.06606138205697221, -5.022037326221688858, -5.474317061061731771 ) ) ;
#21260=ORIENTED_EDGE ( 'NONE', *, *, #16090, .F. ) ;
#21266=AXIS2_PLACEMENT_3D ( 'NONE', #15518, #11418, #19145 ) ;
#21271=EDGE_LOOP ( 'NONE', ( #20709, #3772, #21193, #22936, #13516, #10344, #12732, #12965, #21457, #10664, #5669, #21692, #3063 ) ) ;
#21278=PLANE ( 'NONE',  #23236 ) ;
#21309=AXIS2_PLACEMENT_3D ( 'NONE', #12840, #20691, #10904 ) ;
#21313=ORIENTED_EDGE ( 'NONE', *, *, #11505, .F. ) ;
#21317=FACE_OUTER_BOUND ( 'NONE', #25229, .T. ) ;
#21320=LINE ( 'NONE', #1599, #18506 ) ;
#21331=EDGE_LOOP ( 'NONE', ( #11845, #7360, #24126, #7561 ) ) ;
#21332=ORIENTED_EDGE ( 'NONE', *, *, #22010, .T. ) ;
#21335=CARTESIAN_POINT ( 'NONE',  ( 46.81606138205697221, -3.542416608809818346, -4.744096181734387407 ) ) ;
#21364=ORIENTED_EDGE ( 'NONE', *, *, #20449, .F. ) ;
#21365=CARTESIAN_POINT ( 'NONE',  ( 46.81606138205704326, -28.78650366438485975, 68.66406800134920729 ) ) ;
#21371=AXIS2_PLACEMENT_3D ( 'NONE', #17905, #227, #991 ) ;
#21387=DIRECTION ( 'NONE',  ( -1.225631768639319301E-15, 0.4425581086832399147, -0.8967398287344627850 ) ) ;
#21389=ORIENTED_EDGE ( 'NONE', *, *, #20187, .F. ) ;
#21424=EDGE_LOOP ( 'NONE', ( #22482, #3139, #16701, #9201 ) ) ;
#21430=EDGE_LOOP ( 'NONE', ( #3753, #25166, #9266, #19125, #24225, #16070 ) ) ;
#21441=ORIENTED_EDGE ( 'NONE', *, *, #20519, .T. ) ;
#21451=EDGE_CURVE ( 'NONE', #3268, #19523, #22716, .T. ) ;
#21453=DIRECTION ( 'NONE',  ( -1.000000000000000000, -2.999999999999999839E-15, 0.000000000000000000 ) ) ;
#21457=ORIENTED_EDGE ( 'NONE', *, *, #8071, .T. ) ;
#21478=LINE ( 'NONE', #23143, #21695 ) ;
#21493=ORIENTED_EDGE ( 'NONE', *, *, #15467, .T. ) ;
#21494=CARTESIAN_POINT ( 'NONE',  ( 42.96606138205697789, -6.230354416574639842, -1.331254207427787328 ) ) ;
#21504=AXIS2_PLACEMENT_3D ( 'NONE', #20837, #21214, #13368 ) ;
#21515=VECTOR ( 'NONE', #19745, 1000.000000000000000 ) ;
#21550=CARTESIAN_POINT ( 'NONE',  ( 45.06606138205707879, -39.99575152356565155, 63.13209164280871022 ) ) ;
#21553=FACE_OUTER_BOUND ( 'NONE', #16002, .T. ) ;
#21558=CARTESIAN_POINT ( 'NONE',  ( 44.71606138205694947, 3.586515973360805187, -0.5067327973472466329 ) ) ;
#21560=CARTESIAN_POINT ( 'NONE',  ( 34.81606138205696510, -1.975699482566735776, -4.057200616784870206 ) ) ;
#21578=AXIS2_PLACEMENT_3D ( 'NONE', #18867, #7270, #6885 ) ;
#21591=EDGE_CURVE ( 'NONE', #20374, #20593, #7516, .T. ) ;
#21593=CARTESIAN_POINT ( 'NONE',  ( 45.06606138205697221, -5.022037326221688858, -5.474317061061731771 ) ) ;
#21615=ADVANCED_FACE ( 'NONE', ( #21553 ), #8277, .T. ) ;
#21618=ORIENTED_EDGE ( 'NONE', *, *, #9585, .F. ) ;
#21619=CARTESIAN_POINT ( 'NONE',  ( 29.81606138205705037, -30.46100403034036219, 72.05704881431053366 ) ) ;
#21623=ORIENTED_EDGE ( 'NONE', *, *, #20581, .T. ) ;
#21627=DIRECTION ( 'NONE',  ( -1.000000000000000000, -3.091505625455828697E-15, -4.515976121274772923E-17 ) ) ;
#21634=DIRECTION ( 'NONE',  ( -1.000000000000000000, -2.999999999999999839E-15, 0.000000000000000000 ) ) ;
#21635=CARTESIAN_POINT ( 'NONE',  ( 44.71606138205696368, -0.07962245140794195486, -2.393377716359348817 ) ) ;
#21653=CARTESIAN_POINT ( 'NONE',  ( 29.81606138205707168, -37.70325315460882365, 65.37863370302704880 ) ) ;
#21654=LINE ( 'NONE', #19097, #6739 ) ;
#21658=CARTESIAN_POINT ( 'NONE',  ( 46.81606138205701484, -19.24645833192446176, 25.04281637636312041 ) ) ;
#21668=LINE ( 'NONE', #15989, #4502 ) ;
#21683=VERTEX_POINT ( 'NONE', #9962 ) ;
#21685=DIRECTION ( 'NONE',  ( 0.000000000000000000, -0.8967398287344626739, -0.4425581086832399702 ) ) ;
#21692=ORIENTED_EDGE ( 'NONE', *, *, #3190, .T. ) ;
#21695=VECTOR ( 'NONE', #5517, 1000.000000000000000 ) ;
#21706=EDGE_CURVE ( 'NONE', #5497, #19553, #6347, .T. ) ;
#21713=DIRECTION ( 'NONE',  ( -1.000000000000000000, -2.999999999999999839E-15, 0.000000000000000000 ) ) ;
#21730=VERTEX_POINT ( 'NONE', #9833 ) ;
#21762=CARTESIAN_POINT ( 'NONE',  ( 43.31606138205695089, 3.741517323833267294, 2.753690589366190711 ) ) ;
#21772=ORIENTED_EDGE ( 'NONE', *, *, #7921, .T. ) ;
#21782=CARTESIAN_POINT ( 'NONE',  ( 29.81606138205707168, -36.80651332587436286, 65.82119181171029254 ) ) ;
#21789=CARTESIAN_POINT ( 'NONE',  ( 46.81606138205695800, -0.7562224151693112129, -1.633662118351544734 ) ) ;
#21791=CARTESIAN_POINT ( 'NONE',  ( 33.31606138205697221, -3.118133360756983663, 16.65315793475036443 ) ) ;
#21797=VECTOR ( 'NONE', #15517, 1000.000000000000000 ) ;
#21829=EDGE_CURVE ( 'NONE', #3268, #545, #776, .T. ) ;
#21830=CIRCLE ( 'NONE', #25090, 0.7500000000000001110 ) ;
#21845=CARTESIAN_POINT ( 'NONE',  ( 35.56606138205700063, -13.51824891481310509, 37.72654391001022134 ) ) ;
#21859=VERTEX_POINT ( 'NONE', #5040 ) ;
#21867=PRODUCT_DEFINITION_SHAPE ( 'NONE', 'NONE',  #25194 ) ;
#21874=ORIENTED_EDGE ( 'NONE', *, *, #11159, .T. ) ;
#21904=CIRCLE ( 'NONE', #11639, 4.000000000000000000 ) ;
#21907=FACE_OUTER_BOUND ( 'NONE', #18666, .T. ) ;
#21914=VECTOR ( 'NONE', #480, 1000.000000000000000 ) ;
#21926=EDGE_CURVE ( 'NONE', #23160, #17369, #15918, .T. ) ;
#21938=ORIENTED_EDGE ( 'NONE', *, *, #23090, .T. ) ;
#21945=EDGE_CURVE ( 'NONE', #16500, #22610, #20500, .T. ) ;
#21951=AXIS2_PLACEMENT_3D ( 'NONE', #13967, #4312, #13718 ) ;
#21954=ORIENTED_EDGE ( 'NONE', *, *, #1302, .T. ) ;
#21958=CARTESIAN_POINT ( 'NONE',  ( 41.81606138205696510, -0.1886652901601590937, -3.819484830245897911 ) ) ;
#21964=ORIENTED_EDGE ( 'NONE', *, *, #8608, .F. ) ;
#21983=AXIS2_PLACEMENT_3D ( 'NONE', #18862, #10632, #16535 ) ;
#21991=CARTESIAN_POINT ( 'NONE',  ( 38.31606138205692247, 12.90996180647746350, 7.674666182279729298 ) ) ;
#21993=CARTESIAN_POINT ( 'NONE',  ( 36.31606138205698642, -9.092667827980706718, 28.75914562266559926 ) ) ;
#21994=PLANE ( 'NONE',  #8571 ) ;
#21995=EDGE_CURVE ( 'NONE', #20600, #9497, #12786, .T. ) ;
#21998=EDGE_LOOP ( 'NONE', ( #1918, #8896, #17241, #23100 ) ) ;
#22000=EDGE_LOOP ( 'NONE', ( #17989, #13482, #3148, #10139 ) ) ;
#22009=DIRECTION ( 'NONE',  ( 2.690219486203388234E-15, -0.8967398287344627850, -0.4425581086832399147 ) ) ;
#22010=EDGE_CURVE ( 'NONE', #8578, #18480, #25458, .T. ) ;
#22012=DIRECTION ( 'NONE',  ( -1.327674326049719602E-15, 0.4425581086832399147, -0.8967398287344627850 ) ) ;
#22022=VERTEX_POINT ( 'NONE', #3358 ) ;
#22043=DIRECTION ( 'NONE',  ( -1.000000000000000000, -3.046270958365671426E-15, 5.272995181423179347E-17 ) ) ;
#22053=ORIENTED_EDGE ( 'NONE', *, *, #14281, .F. ) ;
#22057=EDGE_LOOP ( 'NONE', ( #10544, #10015, #9113, #14448 ) ) ;
#22065=DIRECTION ( 'NONE',  ( -1.123589211228918605E-15, 0.4425581086832399147, -0.8967398287344627850 ) ) ;
#22067=ORIENTED_EDGE ( 'NONE', *, *, #17366, .F. ) ;
#22085=CARTESIAN_POINT ( 'NONE',  ( 46.81606138205697221, -3.227578639999799659, -4.500312080287595329 ) ) ;
#22101=DIRECTION ( 'NONE',  ( 1.000000000000000000, 2.954840238787252245E-15, 9.150562545582958565E-17 ) ) ;
#22103=ORIENTED_EDGE ( 'NONE', *, *, #6897, .F. ) ;
#22112=CLOSED_SHELL ( 'NONE', ( #748, #8623, #13848, #3901, #24411, #12962, #6487, #3386, #10005, #11959, #1053, #2558, #10362, #3824, #5850, #9115, #6657, #19963, #14870, #24702, #22861, #14285, #15308, #25100, #1034, #6101, #15009, #4676, #8856, #5958, #20686, #1274, #25293, #3754, #7847, #22323, #24824, #21615, #2130, #16675, #11259, #19434, #2649, #2344, #4778, #7507, #7225, #5003, #22335, #13356, #24975, #6281, #11711, #23743, #2478, #5943, #14115, #19867, #1728, #17959, #20990, #1071, #1160, #8297, #886, #18138, #17289, #15067, #14887, #24034, #749, #1758, #9030, #20573, #11601, #4231, #25285, #18139, #16055, #16722, #7992, #4248, #2762, #1043, #6588, #25306, #13735, #24685, #8488, #17532, #430, #23306, #8303, #18304, #10690, #16188, #25291, #19637, #579, #13838, #15270, #24994 ) ) ;
#22128=CIRCLE ( 'NONE', #8980, 1.000000000000000888 ) ;
#22129=FACE_OUTER_BOUND ( 'NONE', #11539, .T. ) ;
#22132=LINE ( 'NONE', #12366, #21914 ) ;
#22135=( NAMED_UNIT ( * ) SI_UNIT ( $, .STERADIAN. ) SOLID_ANGLE_UNIT ( ) );
#22138=LINE ( 'NONE', #6183, #17239 ) ;
#22151=CARTESIAN_POINT ( 'NONE',  ( 45.81606138205707168, -36.80651332587431313, 65.82119181171029254 ) ) ;
#22161=PLANE ( 'NONE',  #213 ) ;
#22165=AXIS2_PLACEMENT_3D ( 'NONE', #15061, #14941, #22669 ) ;
#22167=EDGE_CURVE ( 'NONE', #2274, #1644, #22138, .T. ) ;
#22169=LINE ( 'NONE', #2449, #2753 ) ;
#22171=AXIS2_PLACEMENT_3D ( 'NONE', #4901, #20489, #9041 ) ;
#22174=DIRECTION ( 'NONE',  ( 2.690219486203388234E-15, -0.8967398287344627850, -0.4425581086832399147 ) ) ;
#22183=CARTESIAN_POINT ( 'NONE',  ( 46.81606138205702194, -20.92507021039837767, 32.39841118875936132 ) ) ;
#22197=VECTOR ( 'NONE', #11417, 1000.000000000000114 ) ;
#22211=FACE_OUTER_BOUND ( 'NONE', #14132, .T. ) ;
#22244=EDGE_LOOP ( 'NONE', ( #19416, #7655, #12692, #24981 ) ) ;
#22245=EDGE_LOOP ( 'NONE', ( #992, #224, #9243, #23649 ) ) ;
#22254=LINE ( 'NONE', #14273, #5429 ) ;
#22260=CARTESIAN_POINT ( 'NONE',  ( 46.81606138205695800, -0.7562224151693112129, -1.633662118351544734 ) ) ;
#22266=AXIS2_PLACEMENT_3D ( 'NONE', #9881, #6260, #23773 ) ;
#22276=DIRECTION ( 'NONE',  ( -1.000000000000000000, -2.999999999999999839E-15, 0.000000000000000000 ) ) ;
#22277=CARTESIAN_POINT ( 'NONE',  ( 41.96606138205694947, 5.208890205473748480, 5.429380561359602453 ) ) ;
#22279=VERTEX_POINT ( 'NONE', #22399 ) ;
#22284=LINE ( 'NONE', #12260, #17278 ) ;
#22302=APPLICATION_CONTEXT ( 'automotive_design' ) ;
#22323=ADVANCED_FACE ( 'NONE', ( #22778 ), #16858, .T. ) ;
#22326=AXIS2_PLACEMENT_3D ( 'NONE', #3538, #1852, #11414 ) ;
#22329=PLANE ( 'NONE',  #17583 ) ;
#22330=VECTOR ( 'NONE', #17104, 1000.000000000000000 ) ;
#22335=ADVANCED_FACE ( 'NONE', ( #22651 ), #12873, .T. ) ;
#22354=VERTEX_POINT ( 'NONE', #18920 ) ;
#22356=PLANE ( 'NONE',  #14161 ) ;
#22359=EDGE_LOOP ( 'NONE', ( #4517, #8374, #14616, #25039 ) ) ;
#22376=ORIENTED_EDGE ( 'NONE', *, *, #20422, .T. ) ;
#22392=DIRECTION ( 'NONE',  ( -1.000000000000000000, -3.091505625455828697E-15, -4.515976121274772923E-17 ) ) ;
#22399=CARTESIAN_POINT ( 'NONE',  ( 33.31606138205700063, -13.43064139120330758, 11.56373968489310755 ) ) ;
#22411=CARTESIAN_POINT ( 'NONE',  ( 36.31606138205702194, -19.58709462196291184, 24.03834292329984379 ) ) ;
#22421=LINE ( 'NONE', #2698, #12722 ) ;
#22426=DIRECTION ( 'NONE',  ( -1.000000000000000000, -2.999999999999999839E-15, 0.000000000000000000 ) ) ;
#22452=EDGE_CURVE ( 'NONE', #22279, #2625, #7323, .T. ) ;
#22467=DIRECTION ( 'NONE',  ( 2.690219486203388234E-15, -0.8967398287344627850, -0.4425581086832399147 ) ) ;
#22477=PLANE ( 'NONE',  #4080 ) ;
#22479=FACE_OUTER_BOUND ( 'NONE', #658, .T. ) ;
#22482=ORIENTED_EDGE ( 'NONE', *, *, #24048, .F. ) ;
#22484=ORIENTED_EDGE ( 'NONE', *, *, #25452, .F. ) ;
#22496=PLANE ( 'NONE',  #19365 ) ;
#22503=AXIS2_PLACEMENT_3D ( 'NONE', #24216, #8794, #2834 ) ;
#22520=LINE ( 'NONE', #10803, #9450 ) ;
#22526=ORIENTED_EDGE ( 'NONE', *, *, #22645, .F. ) ;
#22537=DIRECTION ( 'NONE',  ( 1.000000000000000000, 0.000000000000000000, 0.000000000000000000 ) ) ;
#22547=DIRECTION ( 'NONE',  ( 1.000000000000000000, 2.751104698760144965E-15, -1.228345504986737969E-16 ) ) ;
#22556=CARTESIAN_POINT ( 'NONE',  ( 43.31606138205698642, -7.467730535347520515, -2.778285769174305919 ) ) ;
#22587=PLANE ( 'NONE',  #3695 ) ;
#22590=AXIS2_PLACEMENT_3D ( 'NONE', #8528, #6587, #14447 ) ;
#22596=PLANE ( 'NONE',  #21983 ) ;
#22598=VECTOR ( 'NONE', #5657, 1000.000000000000000 ) ;
#22603=CARTESIAN_POINT ( 'NONE',  ( 46.81606138205706458, -34.55876147768182705, 70.30501292735635843 ) ) ;
#22607=AXIS2_PLACEMENT_3D ( 'NONE', #16583, #22643, #8998 ) ;
#22610=VERTEX_POINT ( 'NONE', #16302 ) ;
#22618=VECTOR ( 'NONE', #5710, 1000.000000000000000 ) ;
#22621=AXIS2_PLACEMENT_3D ( 'NONE', #3731, #2051, #11607 ) ;
#22626=VERTEX_POINT ( 'NONE', #9901 ) ;
#22629=EDGE_CURVE ( 'NONE', #5497, #180, #2022, .T. ) ;
#22643=DIRECTION ( 'NONE',  ( 1.327674326049719602E-15, -0.4425581086832399147, 0.8967398287344627850 ) ) ;
#22645=EDGE_CURVE ( 'NONE', #10246, #19039, #17257, .T. ) ;
#22646=FACE_BOUND ( 'NONE', #6653, .T. ) ;
#22651=FACE_OUTER_BOUND ( 'NONE', #17535, .T. ) ;
#22659=AXIS2_PLACEMENT_3D ( 'NONE', #2899, #16564, #24416 ) ;
#22668=ORIENTED_EDGE ( 'NONE', *, *, #19311, .F. ) ;
#22669=DIRECTION ( 'NONE',  ( -1.000000000000000000, -3.091505625455828697E-15, -4.515976121274772923E-17 ) ) ;
#22704=CARTESIAN_POINT ( 'NONE',  ( 45.81606138205707879, -39.99575152356564445, 63.13209164280871022 ) ) ;
#22716=LINE ( 'NONE', #809, #19629 ) ;
#22719=VERTEX_POINT ( 'NONE', #17887 ) ;
#22736=CARTESIAN_POINT ( 'NONE',  ( 30.81606138205697576, -4.349482454670884124, -5.142398479549302515 ) ) ;
#22744=AXIS2_PLACEMENT_3D ( 'NONE', #21560, #5588, #11277 ) ;
#22750=LINE ( 'NONE', #14638, #23476 ) ;
#22751=ORIENTED_EDGE ( 'NONE', *, *, #2275, .T. ) ;
#22756=VERTEX_POINT ( 'NONE', #214 ) ;
#22760=FACE_OUTER_BOUND ( 'NONE', #2114, .T. ) ;
#22766=CARTESIAN_POINT ( 'NONE',  ( 45.81606138205706458, -34.13844651005145181, 70.48338531520533934 ) ) ;
#22771=DIRECTION ( 'NONE',  ( 1.000000000000000000, 2.611101091812726599E-15, -1.919289851541777660E-16 ) ) ;
#22778=FACE_OUTER_BOUND ( 'NONE', #13167, .T. ) ;
#22782=DIRECTION ( 'NONE',  ( 1.000000000000000000, 2.999999999999999839E-15, 0.000000000000000000 ) ) ;
#22783=ORIENTED_EDGE ( 'NONE', *, *, #25221, .F. ) ;
#22795=CARTESIAN_POINT ( 'NONE',  ( 29.81606138205706458, -34.54722833698622964, 70.28164373264664277 ) ) ;
#22798=DIRECTION ( 'NONE',  ( 2.690219486203388234E-15, -0.8967398287344627850, -0.4425581086832399147 ) ) ;
#22805=CIRCLE ( 'NONE', #14991, 1.499999999999999778 ) ;
#22807=EDGE_CURVE ( 'NONE', #2274, #3431, #15019, .T. ) ;
#22838=AXIS2_PLACEMENT_3D ( 'NONE', #21653, #7628, #23194 ) ;
#22852=ORIENTED_EDGE ( 'NONE', *, *, #24963, .F. ) ;
#22853=DIRECTION ( 'NONE',  ( 1.000000000000000000, 2.999999999999999839E-15, 0.000000000000000000 ) ) ;
#22861=ADVANCED_FACE ( 'NONE', ( #8728 ), #18631, .T. ) ;
#22884=ORIENTED_EDGE ( 'NONE', *, *, #19484, .F. ) ;
#22886=CARTESIAN_POINT ( 'NONE',  ( 29.81606138205706458, -34.54722833698622964, 70.28164373264664277 ) ) ;
#22900=VECTOR ( 'NONE', #20122, 1000.000000000000000 ) ;
#22903=DIRECTION ( 'NONE',  ( 0.000000000000000000, 0.4425581086832397482, -0.8967398287344628960 ) ) ;
#22906=PRODUCT_DEFINITION_CONTEXT ( 'detailed design', #19335, 'design' ) ;
#22913=CARTESIAN_POINT ( 'NONE',  ( 29.81606138205705037, -30.46100403034036219, 72.05704881431053366 ) ) ;
#22936=ORIENTED_EDGE ( 'NONE', *, *, #20684, .T. ) ;
#22939=CARTESIAN_POINT ( 'NONE',  ( 29.81606138205707168, -36.31746077171918330, 73.86860304758450013 ) ) ;
#22949=EDGE_CURVE ( 'NONE', #15873, #22756, #16955, .T. ) ;
#22956=AXIS2_PLACEMENT_3D ( 'NONE', #12092, #13885, #2399 ) ;
#22958=VECTOR ( 'NONE', #5262, 1000.000000000000000 ) ;
#22970=ORIENTED_EDGE ( 'NONE', *, *, #15892, .F. ) ;
#22976=CIRCLE ( 'NONE', #12700, 1.750000000000001776 ) ;
#22983=VECTOR ( 'NONE', #12238, 1000.000000000000000 ) ;
#22985=DIRECTION ( 'NONE',  ( 1.000000000000000000, 2.999999999999999839E-15, 0.000000000000000000 ) ) ;
#22990=VERTEX_POINT ( 'NONE', #9489 ) ;
#22996=EDGE_CURVE ( 'NONE', #19039, #23539, #3424, .T. ) ;
#22998=PLANE ( 'NONE',  #3565 ) ;
#23004=ORIENTED_EDGE ( 'NONE', *, *, #20684, .F. ) ;
#23011=DIRECTION ( 'NONE',  ( 1.000000000000000000, 2.611101091812726599E-15, -1.919289851541777660E-16 ) ) ;
#23012=DIRECTION ( 'NONE',  ( -4.625929269271484533E-15, 0.8967398287344634511, 0.4425581086832385824 ) ) ;
#23027=ORIENTED_EDGE ( 'NONE', *, *, #21829, .T. ) ;
#23039=LINE ( 'NONE', #21365, #12175 ) ;
#23043=ORIENTED_EDGE ( 'NONE', *, *, #24963, .T. ) ;
#23044=DIRECTION ( 'NONE',  ( 1.000000000000000000, 2.999999999999999839E-15, 0.000000000000000000 ) ) ;
#23046=DIRECTION ( 'NONE',  ( 1.000000000000000000, 2.999999999999999839E-15, 0.000000000000000000 ) ) ;
#23048=DIRECTION ( 'NONE',  ( 3.469446951953614189E-15, -0.8967398287344635621, -0.4425581086832386379 ) ) ;
#23067=ORIENTED_EDGE ( 'NONE', *, *, #11473, .F. ) ;
#23088=EDGE_CURVE ( 'NONE', #6472, #10846, #1358, .T. ) ;
#23090=EDGE_CURVE ( 'NONE', #24103, #22354, #21320, .T. ) ;
#23094=ORIENTED_EDGE ( 'NONE', *, *, #15663, .T. ) ;
#23100=ORIENTED_EDGE ( 'NONE', *, *, #24135, .F. ) ;
#23106=EDGE_CURVE ( 'NONE', #1156, #9497, #9621, .T. ) ;
#23107=CARTESIAN_POINT ( 'NONE',  ( 30.81606138205706458, -34.55876147768187678, 70.30501292735635843 ) ) ;
#23111=LINE ( 'NONE', #5727, #18658 ) ;
#23112=CARTESIAN_POINT ( 'NONE',  ( 36.31606138205702194, -19.34838015056931226, 26.94402965816085072 ) ) ;
#23113=AXIS2_PLACEMENT_3D ( 'NONE', #18183, #6075, #10829 ) ;
#23120=EDGE_CURVE ( 'NONE', #23982, #16840, #7803, .T. ) ;
#23130=VERTEX_POINT ( 'NONE', #21080 ) ;
#23131=VERTEX_POINT ( 'NONE', #9246 ) ;
#23138=AXIS2_PLACEMENT_3D ( 'NONE', #16451, #14780, #18906 ) ;
#23142=EDGE_CURVE ( 'NONE', #17733, #559, #10117, .T. ) ;
#23143=CARTESIAN_POINT ( 'NONE',  ( 38.31606138205694378, 2.926944320371558383, 0.2449088955976189141 ) ) ;
#23145=DIRECTION ( 'NONE',  ( -1.000000000000000000, -3.091505625455828697E-15, -4.515976121274772923E-17 ) ) ;
#23148=VECTOR ( 'NONE', #18997, 1000.000000000000000 ) ;
#23150=EDGE_LOOP ( 'NONE', ( #7082, #24476 ) ) ;
#23153=CARTESIAN_POINT ( 'NONE',  ( 45.81606138205707879, -39.99575152356564445, 63.13209164280871022 ) ) ;
#23154=VERTEX_POINT ( 'NONE', #17975 ) ;
#23159=VECTOR ( 'NONE', #2075, 1000.000000000000000 ) ;
#23160=VERTEX_POINT ( 'NONE', #21958 ) ;
#23169=LINE ( 'NONE', #24959, #22598 ) ;
#23176=CARTESIAN_POINT ( 'NONE',  ( 45.81606138205706458, -34.54722833698617990, 70.28164373264664277 ) ) ;
#23184=ORIENTED_EDGE ( 'NONE', *, *, #8727, .F. ) ;
#23193=ORIENTED_EDGE ( 'NONE', *, *, #4215, .F. ) ;
#23194=DIRECTION ( 'NONE',  ( 3.469446951953614189E-15, -0.8967398287344635621, -0.4425581086832386379 ) ) ;
#23203=CARTESIAN_POINT ( 'NONE',  ( 29.81606138205707168, -37.26069504592558701, 64.48189387429259511 ) ) ;
#23205=CARTESIAN_POINT ( 'NONE',  ( 30.81606138205705037, -30.46100403034035509, 72.05704881431053366 ) ) ;
#23219=ORIENTED_EDGE ( 'NONE', *, *, #4337, .F. ) ;
#23220=CARTESIAN_POINT ( 'NONE',  ( 45.06606138205697221, -5.022037326221688858, -5.474317061061731771 ) ) ;
#23221=VECTOR ( 'NONE', #18909, 1000.000000000000000 ) ;
#23228=VERTEX_POINT ( 'NONE', #6244 ) ;
#23236=AXIS2_PLACEMENT_3D ( 'NONE', #21791, #19597, #17295 ) ;
#23244=ORIENTED_EDGE ( 'NONE', *, *, #8071, .F. ) ;
#23246=EDGE_CURVE ( 'NONE', #13742, #545, #5867, .T. ) ;
#23255=DIRECTION ( 'NONE',  ( -1.000000000000000000, -2.999999999999999839E-15, 0.000000000000000000 ) ) ;
#23261=CARTESIAN_POINT ( 'NONE',  ( 39.31606138205697931, -10.17000407126883843, 36.59108960988216808 ) ) ;
#23266=EDGE_CURVE ( 'NONE', #18450, #13333, #20153, .T. ) ;
#23267=CARTESIAN_POINT ( 'NONE',  ( 33.31606138205698642, -7.467730535347551601, -2.778285769174305919 ) ) ;
#23270=EDGE_CURVE ( 'NONE', #16929, #13742, #8057, .T. ) ;
#23273=DIRECTION ( 'NONE',  ( 1.000000000000000000, 2.602085213965208275E-15, 0.000000000000000000 ) ) ;
#23283=EDGE_LOOP ( 'NONE', ( #17605, #12161, #21954, #14593 ) ) ;
#23284=ORIENTED_EDGE ( 'NONE', *, *, #17611, .T. ) ;
#23295=DIRECTION ( 'NONE',  ( 1.000000000000000000, 2.999999999999999839E-15, 0.000000000000000000 ) ) ;
#23296=DIRECTION ( 'NONE',  ( 1.000000000000000000, 2.999999999999999839E-15, 0.000000000000000000 ) ) ;
#23306=ADVANCED_FACE ( 'NONE', ( #4694, #24375 ), #22587, .T. ) ;
#23311=CARTESIAN_POINT ( 'NONE',  ( 40.56606138205696510, -1.522470315718718270, 0.9921758631592225708 ) ) ;
#23351=DIRECTION ( 'NONE',  ( -1.000000000000000000, -3.243061817617045614E-15, -1.199556157213611407E-16 ) ) ;
#23355=DIRECTION ( 'NONE',  ( -2.048868001712896742E-15, 0.6595716529892345914, -0.7516416929448823669 ) ) ;
#23362=CARTESIAN_POINT ( 'NONE',  ( 41.06606138205703616, -24.72749677399387735, 32.19456755146972426 ) ) ;
#23376=ORIENTED_EDGE ( 'NONE', *, *, #15511, .F. ) ;
#23384=CYLINDRICAL_SURFACE ( 'NONE', #1285, 1.500000000000000222 ) ;
#23395=DIRECTION ( 'NONE',  ( -2.048868001712896742E-15, 0.6595716529892345914, -0.7516416929448823669 ) ) ;
#23396=AXIS2_PLACEMENT_3D ( 'NONE', #7471, #19572, #23048 ) ;
#23404=LINE ( 'NONE', #1762, #12380 ) ;
#23434=VECTOR ( 'NONE', #4817, 1000.000000000000000 ) ;
#23437=ORIENTED_EDGE ( 'NONE', *, *, #10660, .F. ) ;
#23454=CARTESIAN_POINT ( 'NONE',  ( 35.56606138205697221, -5.022037326221718168, -5.474317061061731771 ) ) ;
#23459=PLANE ( 'NONE',  #8940 ) ;
#23461=CARTESIAN_POINT ( 'NONE',  ( 43.31606138205700063, -13.43064139120327560, 11.56373968489310755 ) ) ;
#23462=EDGE_CURVE ( 'NONE', #22022, #7686, #21011, .T. ) ;
#23468=DIRECTION ( 'NONE',  ( -1.000000000000000000, -2.999999999999999839E-15, 0.000000000000000000 ) ) ;
#23476=VECTOR ( 'NONE', #4981, 1000.000000000000000 ) ;
#23489=EDGE_CURVE ( 'NONE', #23228, #8670, #17274, .T. ) ;
#23499=DIRECTION ( 'NONE',  ( -1.219254108801168961E-15, 0.4425581086832399147, -0.8967398287344627850 ) ) ;
#23501=ORIENTED_EDGE ( 'NONE', *, *, #19801, .T. ) ;
#23522=ORIENTED_EDGE ( 'NONE', *, *, #15365, .F. ) ;
#23525=DIRECTION ( 'NONE',  ( 1.157642374584902751E-15, -0.3934158747763039088, 0.9193606199277819524 ) ) ;
#23526=CARTESIAN_POINT ( 'NONE',  ( 41.81606138205697221, -3.103162021984027241, -5.046558096268735305 ) ) ;
#23535=DIRECTION ( 'NONE',  ( 1.000000000000000000, 2.805550545906363219E-15, -9.596449257708877207E-17 ) ) ;
#23536=ORIENTED_EDGE ( 'NONE', *, *, #13440, .T. ) ;
#23539=VERTEX_POINT ( 'NONE', #4129 ) ;
#23545=FACE_OUTER_BOUND ( 'NONE', #9854, .T. ) ;
#23549=EDGE_CURVE ( 'NONE', #18450, #12829, #13533, .T. ) ;
#23550=DIRECTION ( 'NONE',  ( 2.792262043613788535E-15, -0.8967398287344627850, -0.4425581086832399147 ) ) ;
#23556=EDGE_CURVE ( 'NONE', #12192, #17722, #17533, .T. ) ;
#23563=ORIENTED_EDGE ( 'NONE', *, *, #10192, .F. ) ;
#23572=VECTOR ( 'NONE', #16804, 1000.000000000000000 ) ;
#23581=DIRECTION ( 'NONE',  ( 1.000000000000000000, 2.751104698760144965E-15, -1.228345504986739201E-16 ) ) ;
#23593=CARTESIAN_POINT ( 'NONE',  ( 37.31606138205702194, -20.92507021039840254, 32.39841118875936132 ) ) ;
#23594=VECTOR ( 'NONE', #17931, 1000.000000000000000 ) ;
#23597=LINE ( 'NONE', #2450, #23159 ) ;
#23606=EDGE_LOOP ( 'NONE', ( #4417, #14917, #18294, #3120 ) ) ;
#23608=EDGE_LOOP ( 'NONE', ( #19625, #21938, #9025, #16376 ) ) ;
#23609=CARTESIAN_POINT ( 'NONE',  ( 30.81606138205696865, -3.227578639999848509, -4.500312080287595329 ) ) ;
#23618=AXIS2_PLACEMENT_3D ( 'NONE', #25079, #7464, #13398 ) ;
#23634=ORIENTED_EDGE ( 'NONE', *, *, #23270, .F. ) ;
#23641=CARTESIAN_POINT ( 'NONE',  ( 31.91606138205697363, -4.349482454670880571, -5.142398479549302515 ) ) ;
#23649=ORIENTED_EDGE ( 'NONE', *, *, #19178, .F. ) ;
#23659=LINE ( 'NONE', #6015, #8824 ) ;
#23663=CARTESIAN_POINT ( 'NONE',  ( 41.06606138205703616, -24.72749677399387380, 32.19456755146972426 ) ) ;
#23669=DIRECTION ( 'NONE',  ( 2.792262043613788535E-15, -0.8967398287344627850, -0.4425581086832398592 ) ) ;
#23671=DIRECTION ( 'NONE',  ( 0.000000000000000000, -0.7516416929448823669, -0.6595716529892345914 ) ) ;
#23677=DIRECTION ( 'NONE',  ( 1.327674326049700866E-15, -0.4425581086832336419, 0.8967398287344658936 ) ) ;
#23684=EDGE_CURVE ( 'NONE', #20897, #4191, #9072, .T. ) ;
#23687=CARTESIAN_POINT ( 'NONE',  ( 45.81606138205705037, -30.65246816789533213, 72.44500581826358143 ) ) ;
#23692=DIRECTION ( 'NONE',  ( -1.000000000000000000, -2.999999999999999839E-15, 0.000000000000000000 ) ) ;
#23702=( NAMED_UNIT ( * ) SI_UNIT ( $, .STERADIAN. ) SOLID_ANGLE_UNIT ( ) );
#23703=ORIENTED_EDGE ( 'NONE', *, *, #714, .T. ) ;
#23711=EDGE_CURVE ( 'NONE', #20407, #20277, #15636, .T. ) ;
#23722=VECTOR ( 'NONE', #1850, 1000.000000000000000 ) ;
#23730=LINE ( 'NONE', #11904, #14475 ) ;
#23737=CARTESIAN_POINT ( 'NONE',  ( 46.81606138205697221, -3.227578639999799659, -4.500312080287595329 ) ) ;
#23742=MECHANICAL_DESIGN_GEOMETRIC_PRESENTATION_REPRESENTATION('',(#9371),#1135);
#23743=ADVANCED_FACE ( 'NONE', ( #16334 ), #12377, .T. ) ;
#23744=ORIENTED_EDGE ( 'NONE', *, *, #18319, .F. ) ;
#23748=CYLINDRICAL_SURFACE ( 'NONE', #21951, 1.750000000000001554 ) ;
#23749=CARTESIAN_POINT ( 'NONE',  ( 40.56606138205697931, -5.948051402551118194, 9.959574150503843981 ) ) ;
#23752=ORIENTED_EDGE ( 'NONE', *, *, #16642, .F. ) ;
#23759=CARTESIAN_POINT ( 'NONE',  ( 31.91606138205697718, -5.918777154956192277, -5.916875169744970187 ) ) ;
#23773=DIRECTION ( 'NONE',  ( -1.000000000000000000, -2.602085213965208275E-15, 0.000000000000000000 ) ) ;
#23780=CARTESIAN_POINT ( 'NONE',  ( 43.31606138205698642, -7.467730535347520515, -2.778285769174305919 ) ) ;
#23783=AXIS2_PLACEMENT_3D ( 'NONE', #14514, #11168, #24665 ) ;
#23786=DIRECTION ( 'NONE',  ( -1.000000000000000000, -2.777772052464415468E-15, 1.096737058023870976E-16 ) ) ;
#23794=AXIS2_PLACEMENT_3D ( 'NONE', #15499, #7409, #19373 ) ;
#23805=DIRECTION ( 'NONE',  ( -1.067465804653198538E-15, 0.4425581086832399147, -0.8967398287344627850 ) ) ;
#23808=FACE_OUTER_BOUND ( 'NONE', #452, .T. ) ;
#23812=VECTOR ( 'NONE', #6971, 1000.000000000000000 ) ;
#23826=CARTESIAN_POINT ( 'NONE',  ( 40.31606138205699352, -10.17000407126883488, 36.59108960988216808 ) ) ;
#23827=DIRECTION ( 'NONE',  ( 1.327674326049719602E-15, -0.4425581086832399147, 0.8967398287344627850 ) ) ;
#23839=VECTOR ( 'NONE', #23692, 1000.000000000000000 ) ;
#23848=ORIENTED_EDGE ( 'NONE', *, *, #21945, .T. ) ;
#23858=CIRCLE ( 'NONE', #12780, 4.000000000000000000 ) ;
#23883=EDGE_LOOP ( 'NONE', ( #11704, #19120, #5905, #15367 ) ) ;
#23903=EDGE_LOOP ( 'NONE', ( #17544, #13911, #115, #13636 ) ) ;
#23922=DIRECTION ( 'NONE',  ( 2.792262043613788535E-15, -0.8967398287344627850, -0.4425581086832399147 ) ) ;
#23930=VECTOR ( 'NONE', #782, 1000.000000000000000 ) ;
#23931=LINE ( 'NONE', #19829, #6283 ) ;
#23940=DIRECTION ( 'NONE',  ( 1.000000000000000000, 3.046345864243081498E-15, 1.366653866685770437E-16 ) ) ;
#23949=EDGE_CURVE ( 'NONE', #17786, #9852, #18790, .T. ) ;
#23951=EDGE_LOOP ( 'NONE', ( #489, #16681 ) ) ;
#23953=DIRECTION ( 'NONE',  ( -1.327674326049719602E-15, 0.4425581086832399147, -0.8967398287344627850 ) ) ;
#23957=DIRECTION ( 'NONE',  ( -2.417197558325568929E-15, 0.6529557272876933549, 0.7573960774932753104 ) ) ;
#23977=ORIENTED_EDGE ( 'NONE', *, *, #7513, .T. ) ;
#23982=VERTEX_POINT ( 'NONE', #867 ) ;
#23989=PLANE ( 'NONE',  #13497 ) ;
#23993=DIRECTION ( 'NONE',  ( 1.000000000000000000, 2.999999999999999839E-15, 0.000000000000000000 ) ) ;
#23999=FACE_OUTER_BOUND ( 'NONE', #22245, .T. ) ;
#24012=EDGE_CURVE ( 'NONE', #17666, #11586, #3193, .T. ) ;
#24016=CARTESIAN_POINT ( 'NONE',  ( 31.56606138205707168, -38.42645682328038248, 63.90656833300437256 ) ) ;
#24021=EDGE_CURVE ( 'NONE', #23154, #18450, #21830, .T. ) ;
#24027=AXIS2_PLACEMENT_3D ( 'NONE', #1578, #24511, #16936 ) ;
#24034=ADVANCED_FACE ( 'NONE', ( #20853 ), #1396, .F. ) ;
#24035=CARTESIAN_POINT ( 'NONE',  ( 30.81606138205707168, -37.70325315460881654, 65.37863370302704880 ) ) ;
#24048=EDGE_CURVE ( 'NONE', #8869, #21859, #6193, .T. ) ;
#24055=LINE ( 'NONE', #4364, #18227 ) ;
#24063=CARTESIAN_POINT ( 'NONE',  ( 45.06606138205697221, -4.349482454670840603, -5.142398479549302515 ) ) ;
#24075=DIRECTION ( 'NONE',  ( -1.000000000000000000, -2.999999999999999839E-15, 0.000000000000000000 ) ) ;
#24077=ORIENTED_EDGE ( 'NONE', *, *, #1820, .T. ) ;
#24091=EDGE_CURVE ( 'NONE', #22, #8257, #23858, .T. ) ;
#24099=ORIENTED_EDGE ( 'NONE', *, *, #8278, .T. ) ;
#24100=LINE ( 'NONE', #22183, #19749 ) ;
#24103=VERTEX_POINT ( 'NONE', #1631 ) ;
#24111=ORIENTED_EDGE ( 'NONE', *, *, #19311, .T. ) ;
#24113=DIRECTION ( 'NONE',  ( 1.000000000000000000, 3.091505625455829092E-15, 4.515976121274730398E-17 ) ) ;
#24123=ORIENTED_EDGE ( 'NONE', *, *, #13505, .F. ) ;
#24125=ORIENTED_EDGE ( 'NONE', *, *, #18080, .F. ) ;
#24126=ORIENTED_EDGE ( 'NONE', *, *, #4207, .T. ) ;
#24135=EDGE_CURVE ( 'NONE', #10246, #20035, #23404, .T. ) ;
#24140=VECTOR ( 'NONE', #18876, 1000.000000000000000 ) ;
#24143=CARTESIAN_POINT ( 'NONE',  ( 36.31606138205702194, -20.02093502212016318, 26.61211107664843212 ) ) ;
#24165=CARTESIAN_POINT ( 'NONE',  ( 29.81606138205707879, -38.42645682328038959, 63.90656833300437256 ) ) ;
#24177=EDGE_CURVE ( 'NONE', #12724, #15674, #13389, .T. ) ;
#24179=EDGE_CURVE ( 'NONE', #14019, #16125, #13765, .T. ) ;
#24182=EDGE_CURVE ( 'NONE', #21730, #2758, #17757, .T. ) ;
#24187=ORIENTED_EDGE ( 'NONE', *, *, #17022, .T. ) ;
#24194=FACE_OUTER_BOUND ( 'NONE', #25286, .T. ) ;
#24198=CARTESIAN_POINT ( 'NONE',  ( 31.56606138205697576, -4.349482454670882348, -5.142398479549302515 ) ) ;
#24211=VERTEX_POINT ( 'NONE', #2024 ) ;
#24212=PLANE ( 'NONE',  #13151 ) ;
#24216=CARTESIAN_POINT ( 'NONE',  ( 41.81606138205696510, -1.316127829577467656, -4.808842309729777220 ) ) ;
#24218=ORIENTED_EDGE ( 'NONE', *, *, #5989, .F. ) ;
#24220=ORIENTED_EDGE ( 'NONE', *, *, #18399, .T. ) ;
#24222=CARTESIAN_POINT ( 'NONE',  ( 31.91606138205697718, -5.022037326221728826, -5.474317061061731771 ) ) ;
#24225=ORIENTED_EDGE ( 'NONE', *, *, #20519, .F. ) ;
#24235=EDGE_CURVE ( 'NONE', #13201, #22354, #4605, .T. ) ;
#24236=AXIS2_PLACEMENT_3D ( 'NONE', #19677, #20188, #23671 ) ;
#24240=VECTOR ( 'NONE', #1935, 1000.000000000000000 ) ;
#24252=AXIS2_PLACEMENT_3D ( 'NONE', #11903, #15370, #5587 ) ;
#24256=DIRECTION ( 'NONE',  ( -1.000000000000000000, -2.999999999999999839E-15, 0.000000000000000000 ) ) ;
#24276=ORIENTED_EDGE ( 'NONE', *, *, #13045, .T. ) ;
#24281=DIRECTION ( 'NONE',  ( -1.327674326049719602E-15, 0.4425581086832399147, -0.8967398287344627850 ) ) ;
#24287=CARTESIAN_POINT ( 'NONE',  ( 29.81606138205697576, -4.349482454670887677, -5.142398479549302515 ) ) ;
#24288=ORIENTED_EDGE ( 'NONE', *, *, #9648, .F. ) ;
#24354=CIRCLE ( 'NONE', #5866, 0.7500000000000001110 ) ;
#24375=FACE_OUTER_BOUND ( 'NONE', #24973, .T. ) ;
#24392=PLANE ( 'NONE',  #5528 ) ;
#24397=DIRECTION ( 'NONE',  ( -1.327674326049719602E-15, 0.4425581086832399147, -0.8967398287344627850 ) ) ;
#24411=ADVANCED_FACE ( 'NONE', ( #20568 ), #22496, .F. ) ;
#24414=EDGE_CURVE ( 'NONE', #23539, #20035, #1269, .T. ) ;
#24416=DIRECTION ( 'NONE',  ( 0.000000000000000000, -0.7516416929448823669, -0.6595716529892345914 ) ) ;
#24429=EDGE_CURVE ( 'NONE', #17110, #3839, #22750, .T. ) ;
#24443=CARTESIAN_POINT ( 'NONE',  ( 40.56606138205695089, 2.967040633637585856, 4.322985289651505525 ) ) ;
#24444=EDGE_LOOP ( 'NONE', ( #18382, #25183, #14662, #645 ) ) ;
#24449=DIRECTION ( 'NONE',  ( 1.000000000000000000, 2.999999999999999839E-15, 0.000000000000000000 ) ) ;
#24457=DIRECTION ( 'NONE',  ( -2.048868001712896742E-15, 0.6595716529892345914, -0.7516416929448823669 ) ) ;
#24468=CARTESIAN_POINT ( 'NONE',  ( 40.31606138205702194, -20.80831168696338196, 24.25326155172387033 ) ) ;
#24476=ORIENTED_EDGE ( 'NONE', *, *, #24414, .F. ) ;
#24511=DIRECTION ( 'NONE',  ( -1.000000000000000000, -3.046345864243081498E-15, -1.366653866685770437E-16 ) ) ;
#24517=EDGE_CURVE ( 'NONE', #20166, #5217, #19022, .T. ) ;
#24521=ORIENTED_EDGE ( 'NONE', *, *, #16717, .T. ) ;
#24531=CARTESIAN_POINT ( 'NONE',  ( 46.81606138205695800, -0.7562224151693112129, -1.633662118351544734 ) ) ;
#24534=AXIS2_PLACEMENT_3D ( 'NONE', #13470, #3666, #19521 ) ;
#24549=CARTESIAN_POINT ( 'NONE',  ( 37.31606138205702194, -21.37925193044963024, 31.05911325134166034 ) ) ;
#24569=DIRECTION ( 'NONE',  ( -2.048868001712896742E-15, 0.6595716529892345914, -0.7516416929448823669 ) ) ;
#24570=ORIENTED_EDGE ( 'NONE', *, *, #16717, .F. ) ;
#24576=DIRECTION ( 'NONE',  ( 0.000000000000000000, -0.8967398287344634511, -0.4425581086832385824 ) ) ;
#24579=EDGE_CURVE ( 'NONE', #13632, #4703, #3429, .T. ) ;
#24587=AXIS2_PLACEMENT_3D ( 'NONE', #14263, #23786, #20186 ) ;
#24589=CARTESIAN_POINT ( 'NONE',  ( 31.56606138205707879, -39.99575152356569419, 63.13209164280871022 ) ) ;
#24600=VECTOR ( 'NONE', #16472, 1000.000000000000000 ) ;
#24604=DIRECTION ( 'NONE',  ( 0.000000000000000000, -0.8967398287344635621, -0.4425581086832386379 ) ) ;
#24606=FACE_OUTER_BOUND ( 'NONE', #17221, .T. ) ;
#24608=CARTESIAN_POINT ( 'NONE',  ( 41.06606138205700063, -13.51824891481308910, 37.72654391001022134 ) ) ;
#24611=CARTESIAN_POINT ( 'NONE',  ( 43.31606138205697221, -3.118133360756952577, 16.65315793475036443 ) ) ;
#24622=AXIS2_PLACEMENT_3D ( 'NONE', #14676, #22798, #5158 ) ;
#24637=CARTESIAN_POINT ( 'NONE',  ( 29.81606138205707879, -39.99575152356569419, 63.13209164280871022 ) ) ;
#24638=ORIENTED_EDGE ( 'NONE', *, *, #24021, .T. ) ;
#24645=CARTESIAN_POINT ( 'NONE',  ( 31.91606138205695231, 3.586515973360766996, -0.5067327973472466329 ) ) ;
#24647=ORIENTED_EDGE ( 'NONE', *, *, #24091, .F. ) ;
#24657=VECTOR ( 'NONE', #1366, 1000.000000000000000 ) ;
#24665=DIRECTION ( 'NONE',  ( -1.327674326049719602E-15, 0.4425581086832399147, -0.8967398287344627850 ) ) ;
#24676=LINE ( 'NONE', #10923, #22330 ) ;
#24679=VECTOR ( 'NONE', #4786, 1000.000000000000000 ) ;
#24685=ADVANCED_FACE ( 'NONE', ( #5871 ), #21083, .T. ) ;
#24699=UNCERTAINTY_MEASURE_WITH_UNIT (LENGTH_MEASURE( 1.000000000000000082E-05 ), #5109, 'distance_accuracy_value', 'NONE');
#24702=ADVANCED_FACE ( 'NONE', ( #11421 ), #19267, .T. ) ;
#24710=LINE ( 'NONE', #7084, #345 ) ;
#24735=ORIENTED_EDGE ( 'NONE', *, *, #23949, .F. ) ;
#24741=DIRECTION ( 'NONE',  ( 2.690219486203388234E-15, -0.8967398287344627850, -0.4425581086832399147 ) ) ;
#24744=EDGE_CURVE ( 'NONE', #23130, #17110, #10752, .T. ) ;
#24749=VECTOR ( 'NONE', #17548, 1000.000000000000000 ) ;
#24761=ORIENTED_EDGE ( 'NONE', *, *, #7513, .F. ) ;
#24767=LINE ( 'NONE', #1076, #17465 ) ;
#24773=DIRECTION ( 'NONE',  ( 1.327674326049719602E-15, -0.4425581086832399147, 0.8967398287344627850 ) ) ;
#24783=FILL_AREA_STYLE ('',( #16208 ) ) ;
#24797=CARTESIAN_POINT ( 'NONE',  ( 41.96606138205694236, 6.105630034208208379, 5.871938670042847974 ) ) ;
#24804=ORIENTED_EDGE ( 'NONE', *, *, #11460, .F. ) ;
#24824=ADVANCED_FACE ( 'NONE', ( #22211 ), #433, .F. ) ;
#24832=LINE ( 'NONE', #17249, #23930 ) ;
#24840=EDGE_CURVE ( 'NONE', #5343, #22990, #561, .T. ) ;
#24841=VERTEX_POINT ( 'NONE', #23759 ) ;
#24865=VERTEX_POINT ( 'NONE', #14359 ) ;
#24889=ORIENTED_EDGE ( 'NONE', *, *, #22949, .T. ) ;
#24893=EDGE_LOOP ( 'NONE', ( #5944, #22067, #6069, #20440 ) ) ;
#24896=CARTESIAN_POINT ( 'NONE',  ( 35.56606138205703616, -24.72749677399389157, 32.19456755146972426 ) ) ;
#24899=EDGE_CURVE ( 'NONE', #14345, #16500, #19277, .T. ) ;
#24900=ORIENTED_EDGE ( 'NONE', *, *, #19484, .T. ) ;
#24905=PLANE ( 'NONE',  #22326 ) ;
#24907=CARTESIAN_POINT ( 'NONE',  ( 31.91606138205692389, 12.25039015348819582, 8.426307875224583910 ) ) ;
#24909=CARTESIAN_POINT ( 'NONE',  ( 31.56606138205697576, -4.349482454670882348, -5.142398479549302515 ) ) ;
#24928=ORIENTED_EDGE ( 'NONE', *, *, #15865, .F. ) ;
#24942=VERTEX_POINT ( 'NONE', #7308 ) ;
#24954=ORIENTED_EDGE ( 'NONE', *, *, #19017, .T. ) ;
#24956=CARTESIAN_POINT ( 'NONE',  ( 30.81606138205707524, -38.13418765192407989, 68.51141129791366780 ) ) ;
#24959=CARTESIAN_POINT ( 'NONE',  ( 46.81606138205705747, -33.21365173458013231, 70.96885009038120984 ) ) ;
#24962=EDGE_CURVE ( 'NONE', #58, #13895, #14457, .T. ) ;
#24963=EDGE_CURVE ( 'NONE', #22626, #1156, #1374, .T. ) ;
#24973=EDGE_LOOP ( 'NONE', ( #23563, #10922, #17285, #17703, #1443, #18680, #13233, #6352, #6375, #15793, #22970, #21052, #14518 ) ) ;
#24974=VECTOR ( 'NONE', #16735, 1000.000000000000000 ) ;
#24975=ADVANCED_FACE ( 'NONE', ( #3555 ), #11435, .T. ) ;
#24981=ORIENTED_EDGE ( 'NONE', *, *, #20401, .F. ) ;
#24994=ADVANCED_FACE ( 'NONE', ( #1615 ), #23384, .F. ) ;
#24997=DIRECTION ( 'NONE',  ( 1.734723475976807094E-15, -0.7516416929448819229, -0.6595716529892350355 ) ) ;
#25009=EDGE_LOOP ( 'NONE', ( #6059, #21121, #7404, #25476 ) ) ;
#25017=PLANE ( 'NONE',  #24027 ) ;
#25037=EDGE_LOOP ( 'NONE', ( #315, #4627, #4007, #6790 ) ) ;
#25039=ORIENTED_EDGE ( 'NONE', *, *, #4430, .F. ) ;
#25040=ORIENTED_EDGE ( 'NONE', *, *, #21995, .F. ) ;
#25069=ORIENTED_EDGE ( 'NONE', *, *, #19399, .T. ) ;
#25072=AXIS2_PLACEMENT_3D ( 'NONE', #14702, #12918, #16637 ) ;
#25077=ORIENTED_EDGE ( 'NONE', *, *, #12906, .T. ) ;
#25079=CARTESIAN_POINT ( 'NONE',  ( 36.31606138205701484, -18.91453975041206093, 24.37026150481227305 ) ) ;
#25090=AXIS2_PLACEMENT_3D ( 'NONE', #8757, #22782, #22903 ) ;
#25100=ADVANCED_FACE ( 'NONE', ( #19660 ), #319, .T. ) ;
#25107=SURFACE_SIDE_STYLE ('',( #3493 ) ) ;
#25117=DIRECTION ( 'NONE',  ( 1.000000000000000000, 3.469446951953611033E-15, 0.000000000000000000 ) ) ;
#25121=DIRECTION ( 'NONE',  ( -1.000000000000000000, -2.870367030604242092E-15, 6.397632838472598363E-17 ) ) ;
#25146=CARTESIAN_POINT ( 'NONE',  ( 38.31606138205692247, 12.25039015348821358, 8.426307875224583910 ) ) ;
#25161=DIRECTION ( 'NONE',  ( 1.000000000000000000, 2.751104698760144965E-15, -1.228345504986737969E-16 ) ) ;
#25165=CARTESIAN_POINT ( 'NONE',  ( 29.81606138205696155, -0.7562224151693598406, -1.633662118351544734 ) ) ;
#25166=ORIENTED_EDGE ( 'NONE', *, *, #509, .T. ) ;
#25174=ORIENTED_EDGE ( 'NONE', *, *, #21926, .F. ) ;
#25183=ORIENTED_EDGE ( 'NONE', *, *, #3996, .F. ) ;
#25190=LINE ( 'NONE', #13627, #14498 ) ;
#25193=CARTESIAN_POINT ( 'NONE',  ( 30.81606138205696865, -2.286980848581618986, -4.124514829577853980 ) ) ;
#25194=PRODUCT_DEFINITION ( 'UNKNOWN', '', #5540, #22906 ) ;
#25198=AXIS2_PLACEMENT_3D ( 'NONE', #8721, #12837, #4596 ) ;
#25213=AXIS2_PLACEMENT_3D ( 'NONE', #24198, #23827, #18052 ) ;
#25217=DIRECTION ( 'NONE',  ( 0.000000000000000000, -0.4425581086832400812, 0.8967398287344626739 ) ) ;
#25221=EDGE_CURVE ( 'NONE', #13157, #18170, #12587, .T. ) ;
#25225=CIRCLE ( 'NONE', #20734, 1.750000000000000222 ) ;
#25229=EDGE_LOOP ( 'NONE', ( #14629, #10100, #279, #22484 ) ) ;
#25230=CARTESIAN_POINT ( 'NONE',  ( 29.81606138205697931, -5.918777154956199382, -5.916875169744970187 ) ) ;
#25255=LINE ( 'NONE', #3505, #9791 ) ;
#25269=ORIENTED_EDGE ( 'NONE', *, *, #8001, .T. ) ;
#25281=CARTESIAN_POINT ( 'NONE',  ( 41.81606138205696510, -1.975699482566714904, -4.057200616784870206 ) ) ;
#25283=CIRCLE ( 'NONE', #8865, 1.500000000000000222 ) ;
#25285=ADVANCED_FACE ( 'NONE', ( #14622 ), #22477, .T. ) ;
#25286=EDGE_LOOP ( 'NONE', ( #18328, #18231, #18253, #19148 ) ) ;
#25291=ADVANCED_FACE ( 'NONE', ( #13212 ), #1706, .T. ) ;
#25293=ADVANCED_FACE ( 'NONE', ( #13337, #11402, #15003 ), #9228, .F. ) ;
#25294=EDGE_CURVE ( 'NONE', #23130, #8686, #7152, .T. ) ;
#25306=ADVANCED_FACE ( 'NONE', ( #19128 ), #1469, .T. ) ;
#25307=CARTESIAN_POINT ( 'NONE',  ( 40.31606138205701484, -18.91453975041205382, 24.37026150481227305 ) ) ;
#25313=DIRECTION ( 'NONE',  ( 2.048868001712898319E-15, -0.6595716529892350355, 0.7516416929448821449 ) ) ;
#25315=DIRECTION ( 'NONE',  ( 0.000000000000000000, -0.4425581086832400812, 0.8967398287344626739 ) ) ;
#25317=DIRECTION ( 'NONE',  ( 1.000000000000000000, 2.999999999999999839E-15, 0.000000000000000000 ) ) ;
#25334=ORIENTED_EDGE ( 'NONE', *, *, #19266, .T. ) ;
#25343=ORIENTED_EDGE ( 'NONE', *, *, #8624, .F. ) ;
#25345=LINE ( 'NONE', #1904, #12342 ) ;
#25351=CARTESIAN_POINT ( 'NONE',  ( 33.66606138205694521, 5.208890205473720059, 5.429380561359602453 ) ) ;
#25378=CARTESIAN_POINT ( 'NONE',  ( 40.31606138205702194, -20.48251210171515879, 31.50167136002490764 ) ) ;
#25379=DIRECTION ( 'NONE',  ( -2.545659196538654441E-15, 0.8967398287344627850, 0.4425581086832399147 ) ) ;
#25394=CYLINDRICAL_SURFACE ( 'NONE', #24252, 3.999999999999999556 ) ;
#25404=VECTOR ( 'NONE', #20784, 1000.000000000000000 ) ;
#25417=PLANE ( 'NONE',  #7376 ) ;
#25421=ORIENTED_EDGE ( 'NONE', *, *, #3442, .T. ) ;
#25441=VECTOR ( 'NONE', #9603, 1000.000000000000000 ) ;
#25443=DIRECTION ( 'NONE',  ( -2.312964634635742267E-15, 0.8967398287344626739, 0.4425581086832399147 ) ) ;
#25452=EDGE_CURVE ( 'NONE', #21232, #20277, #18425, .T. ) ;
#25453=CARTESIAN_POINT ( 'NONE',  ( 46.81606138205705037, -30.46100403034031245, 72.05704881431053366 ) ) ;
#25456=FACE_BOUND ( 'NONE', #14608, .T. ) ;
#25458=CIRCLE ( 'NONE', #14771, 3.000000000000000444 ) ;
#25463=EDGE_LOOP ( 'NONE', ( #4888, #19161 ) ) ;
#25469=EDGE_CURVE ( 'NONE', #21232, #12198, #18177, .T. ) ;
#25470=AXIS2_PLACEMENT_3D ( 'NONE', #3851, #11348, #25217 ) ;
#25473=CARTESIAN_POINT ( 'NONE',  ( 36.31606138205703616, -24.57005561077093247, 31.87555009596680478 ) ) ;
#25476=ORIENTED_EDGE ( 'NONE', *, *, #6030, .F. ) ;
#25483=VECTOR ( 'NONE', #19836, 1000.000000000000000 ) ;
ENDSEC;
END-ISO-10303-21;
